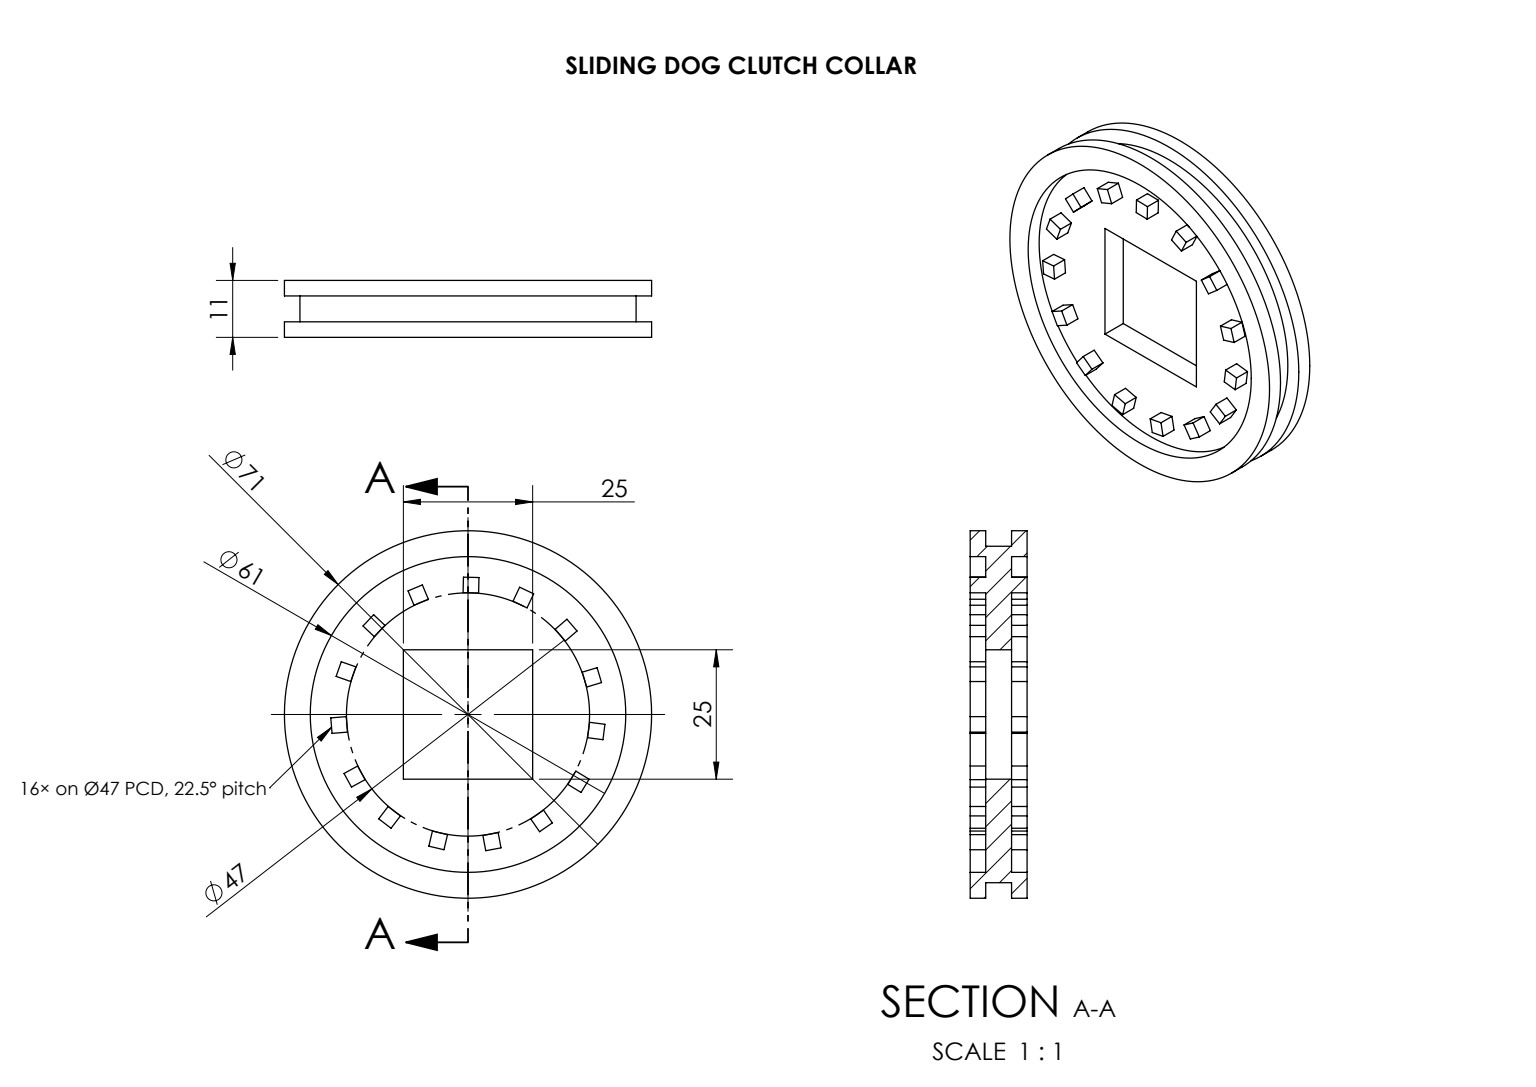
ISO-10303-21;
HEADER;
FILE_DESCRIPTION (('STEP AP214'),
    '1' );
FILE_NAME ('Sliding Dog Clutch Collar.step',
    '2026-09-30T12:41:04',
    ( '' ),
    ( '' ),
    'SwSTEP 2.0',
    'SolidWorks 2026',
    '' );
FILE_SCHEMA (( 'AUTOMOTIVE_DESIGN' ));
ENDSEC;

DATA;
#8=ORIENTED_EDGE ( 'NONE', *, *, #47564, .F. ) ;
#9=CARTESIAN_POINT ( 'NONE',  ( 0.000000000000000000, -120.0000000000000000, -5.500000000000000000 ) ) ;
#30=DIRECTION ( 'NONE',  ( -0.6516173805718067369, 0.7585478161175716050, 0.000000000000000000 ) ) ;
#32=AXIS2_PLACEMENT_3D ( 'NONE', #39036, #42465, #12856 ) ;
#46=EDGE_CURVE ( 'NONE', #39583, #27608, #108, .T. ) ;
#61=VECTOR ( 'NONE', #12342, 1000.000000000000114 ) ;
#65=DIRECTION ( 'NONE',  ( 0.000000000000000000, 1.000000000000000000, 0.000000000000000000 ) ) ;
#66=DIRECTION ( 'NONE',  ( -0.000000000000000000, -0.000000000000000000, -1.000000000000000000 ) ) ;
#75=AXIS2_PLACEMENT_3D ( 'NONE', #43340, #46778, #40148 ) ;
#80=ORIENTED_EDGE ( 'NONE', *, *, #29393, .F. ) ;
#108=LINE ( 'NONE', #14814, #16119 ) ;
#110=FACE_OUTER_BOUND ( 'NONE', #38176, .T. ) ;
#122=CARTESIAN_POINT ( 'NONE',  ( 23.49916127795269460, -121.5130826919798039, -5.500000000000000000 ) ) ;
#149=ORIENTED_EDGE ( 'NONE', *, *, #40004, .F. ) ;
#160=EDGE_CURVE ( 'NONE', #47761, #19570, #831, .T. ) ;
#163=LINE ( 'NONE', #8479, #41980 ) ;
#164=DIRECTION ( 'NONE',  ( -0.9966891607226785466, -0.08130631524010122069, 0.000000000000000000 ) ) ;
#165=CARTESIAN_POINT ( 'NONE',  ( 9.984461079971730157, -95.40710393340120277, 5.500000000000000000 ) ) ;
#171=LINE ( 'NONE', #44725, #4221 ) ;
#173=AXIS2_PLACEMENT_3D ( 'NONE', #10404, #35866, #3285 ) ;
#181=ORIENTED_EDGE ( 'NONE', *, *, #17068, .F. ) ;
#187=EDGE_CURVE ( 'NONE', #17280, #1537, #37135, .T. ) ;
#211=CARTESIAN_POINT ( 'NONE',  ( 21.85433023846371370, -135.0628101570779620, 5.500000000000000000 ) ) ;
#212=CARTESIAN_POINT ( 'NONE',  ( 0.4301293587033142574, -121.4370068666438556, 2.500000000000000000 ) ) ;
#222=CARTESIAN_POINT ( 'NONE',  ( -8.826826895187510402, -94.96827758698185562, 5.500000000000000000 ) ) ;
#244=VECTOR ( 'NONE', #1818, 1000.000000000000114 ) ;
#254=EDGE_LOOP ( 'NONE', ( #41035, #46518, #11215, #569 ) ) ;
#256=VECTOR ( 'NONE', #6458, 1000.000000000000000 ) ;
#273=DIRECTION ( 'NONE',  ( -0.6064928550163533050, -0.7950889364178781449, 0.000000000000000000 ) ) ;
#283=DIRECTION ( 'NONE',  ( -0.3853207896976533764, 0.9227826878668546895, 0.000000000000000000 ) ) ;
#285=VECTOR ( 'NONE', #16064, 1000.000000000000114 ) ;
#296=VECTOR ( 'NONE', #11332, 1000.000000000000227 ) ;
#303=ORIENTED_EDGE ( 'NONE', *, *, #45962, .F. ) ;
#309=DIRECTION ( 'NONE',  ( 0.8774505977381978905, 0.4796670183876304283, 0.000000000000000000 ) ) ;
#324=VECTOR ( 'NONE', #48391, 1000.000000000000114 ) ;
#327=CARTESIAN_POINT ( 'NONE',  ( 21.07894319797337701, -103.8699611390234878, 5.500000000000000000 ) ) ;
#342=CARTESIAN_POINT ( 'NONE',  ( -12.50000000000000000, -107.5000000000000000, 2.500000000000000000 ) ) ;
#355=DIRECTION ( 'NONE',  ( 0.8541291221503275466, -0.5200609990132993854, 0.000000000000000000 ) ) ;
#370=CARTESIAN_POINT ( 'NONE',  ( 12.13205353604972991, -140.1820037904669789, 5.500000000000000000 ) ) ;
#385=ADVANCED_FACE ( 'NONE', ( #12022 ), #4437, .F. ) ;
#392=ORIENTED_EDGE ( 'NONE', *, *, #17689, .T. ) ;
#397=FACE_OUTER_BOUND ( 'NONE', #27506, .T. ) ;
#412=VECTOR ( 'NONE', #23395, 1000.000000000000000 ) ;
#446=CARTESIAN_POINT ( 'NONE',  ( -13.05994868825747446, -139.5943292883446532, 5.500000000000000000 ) ) ;
#448=DIRECTION ( 'NONE',  ( -0.000000000000000000, -0.000000000000000000, -1.000000000000000000 ) ) ;
#449=ORIENTED_EDGE ( 'NONE', *, *, #48116, .F. ) ;
#454=FACE_OUTER_BOUND ( 'NONE', #32688, .T. ) ;
#459=VECTOR ( 'NONE', #14578, 1000.000000000000114 ) ;
#460=ORIENTED_EDGE ( 'NONE', *, *, #19536, .T. ) ;
#473=DIRECTION ( 'NONE',  ( -0.000000000000000000, -0.000000000000000000, -1.000000000000000000 ) ) ;
#474=ORIENTED_EDGE ( 'NONE', *, *, #31629, .F. ) ;
#480=PLANE ( 'NONE',  #23178 ) ;
#482=ORIENTED_EDGE ( 'NONE', *, *, #3297, .T. ) ;
#494=LINE ( 'NONE', #44786, #14354 ) ;
#509=FACE_OUTER_BOUND ( 'NONE', #15713, .T. ) ;
#513=ORIENTED_EDGE ( 'NONE', *, *, #3767, .F. ) ;
#537=DIRECTION ( 'NONE',  ( -0.9730327541852497042, 0.2306669878475622604, 0.000000000000000000 ) ) ;
#542=DIRECTION ( 'NONE',  ( -0.000000000000000000, -0.000000000000000000, -1.000000000000000000 ) ) ;
#544=DIRECTION ( 'NONE',  ( 0.9918136447140100120, -0.1276937514489704939, 0.000000000000000000 ) ) ;
#551=VERTEX_POINT ( 'NONE', #27927 ) ;
#555=EDGE_CURVE ( 'NONE', #16750, #43974, #5886, .T. ) ;
#567=LINE ( 'NONE', #45118, #45725 ) ;
#569=ORIENTED_EDGE ( 'NONE', *, *, #23324, .F. ) ;
#570=CARTESIAN_POINT ( 'NONE',  ( 16.30584220631899228, -140.9432449716519784, 5.500000000000000000 ) ) ;
#571=CARTESIAN_POINT ( 'NONE',  ( 1.029419772574596825, -118.9089936151275140, 2.500000000000000000 ) ) ;
#576=ORIENTED_EDGE ( 'NONE', *, *, #44143, .F. ) ;
#594=LINE ( 'NONE', #15524, #29851 ) ;
#598=CARTESIAN_POINT ( 'NONE',  ( 4.903647372192503795, -146.0423547792665886, 2.500000000000000000 ) ) ;
#601=CARTESIAN_POINT ( 'NONE',  ( 20.85212586905262100, -130.9402397935870965, 5.500000000000000000 ) ) ;
#622=EDGE_LOOP ( 'NONE', ( #38651, #1089, #2965, #8815 ) ) ;
#639=PLANE ( 'NONE',  #10239 ) ;
#656=PLANE ( 'NONE',  #42750 ) ;
#669=ORIENTED_EDGE ( 'NONE', *, *, #7293, .T. ) ;
#693=PLANE ( 'NONE',  #5618 ) ;
#722=LINE ( 'NONE', #11518, #33116 ) ;
#724=ORIENTED_EDGE ( 'NONE', *, *, #41620, .T. ) ;
#730=CARTESIAN_POINT ( 'NONE',  ( 20.85212586905262100, -130.9402397935870965, 2.500000000000000000 ) ) ;
#733=CARTESIAN_POINT ( 'NONE',  ( -23.30023580412278505, -123.4057321492263384, -5.500000000000000000 ) ) ;
#741=FACE_OUTER_BOUND ( 'NONE', #31676, .T. ) ;
#744=ORIENTED_EDGE ( 'NONE', *, *, #10469, .F. ) ;
#748=CARTESIAN_POINT ( 'NONE',  ( -7.572224309238338336, -145.4393675041377492, 5.500000000000000000 ) ) ;
#756=EDGE_CURVE ( 'NONE', #40958, #16750, #45009, .T. ) ;
#769=CARTESIAN_POINT ( 'NONE',  ( -13.05994868825747446, -139.5943292883446532, 5.500000000000000000 ) ) ;
#781=EDGE_LOOP ( 'NONE', ( #17034, #22607, #22558, #21129 ) ) ;
#792=CARTESIAN_POINT ( 'NONE',  ( 0.1219594728601484379, -121.4950337410840149, 2.500000000000000000 ) ) ;
#831=LINE ( 'NONE', #10898, #11447 ) ;
#864=CARTESIAN_POINT ( 'NONE',  ( -14.87942725330654348, -141.9795960975983178, 5.500000000000000000 ) ) ;
#866=LINE ( 'NONE', #30749, #3355 ) ;
#877=AXIS2_PLACEMENT_3D ( 'NONE', #15679, #17351, #43081 ) ;
#896=CARTESIAN_POINT ( 'NONE',  ( -10.43921258969510824, -98.89258801967538659, 5.500000000000000000 ) ) ;
#906=DIRECTION ( 'NONE',  ( 0.5200609990133008287, 0.8541291221503266584, -0.000000000000000000 ) ) ;
#935=CARTESIAN_POINT ( 'NONE',  ( -15.44521549751111422, -137.7748507232956001, 2.500000000000000000 ) ) ;
#974=VECTOR ( 'NONE', #38147, 1000.000000000000000 ) ;
#1021=CARTESIAN_POINT ( 'NONE',  ( 19.29194287201271862, -133.5026271600380880, -5.500000000000000000 ) ) ;
#1026=DIRECTION ( 'NONE',  ( -0.000000000000000000, -0.000000000000000000, -1.000000000000000000 ) ) ;
#1068=VECTOR ( 'NONE', #42092, 1000.000000000000000 ) ;
#1072=VECTOR ( 'NONE', #42654, 1000.000000000000000 ) ;
#1074=ORIENTED_EDGE ( 'NONE', *, *, #30261, .F. ) ;
#1087=ADVANCED_FACE ( 'NONE', ( #43978, #17297, #32251, #21211, #40330, #14365, #36627, #36147, #6784, #21706, #21939, #17545, #3091, #47414, #18018, #47170, #44228 ), #2603, .F. ) ;
#1089=ORIENTED_EDGE ( 'NONE', *, *, #1604, .T. ) ;
#1090=EDGE_CURVE ( 'NONE', #29594, #25561, #7011, .T. ) ;
#1103=ADVANCED_FACE ( 'NONE', ( #30272 ), #41519, .T. ) ;
#1105=CARTESIAN_POINT ( 'NONE',  ( -1.459549131277904976, -119.6539995182286304, 2.500000000000000000 ) ) ;
#1110=DIRECTION ( 'NONE',  ( 0.9997280174009349762, -0.02332147558787674158, 0.000000000000000000 ) ) ;
#1113=CARTESIAN_POINT ( 'NONE',  ( 2.874421927457452952, -143.3717286177755739, 5.500000000000000000 ) ) ;
#1124=AXIS2_PLACEMENT_3D ( 'NONE', #13235, #28158, #27444 ) ;
#1129=AXIS2_PLACEMENT_3D ( 'NONE', #7232, #11155, #3564 ) ;
#1132=VECTOR ( 'NONE', #38496, 1000.000000000000000 ) ;
#1140=ORIENTED_EDGE ( 'NONE', *, *, #8337, .F. ) ;
#1141=AXIS2_PLACEMENT_3D ( 'NONE', #1935, #20508, #43039 ) ;
#1148=EDGE_CURVE ( 'NONE', #30085, #18493, #4073, .T. ) ;
#1152=ORIENTED_EDGE ( 'NONE', *, *, #6211, .T. ) ;
#1157=AXIS2_PLACEMENT_3D ( 'NONE', #25787, #14062, #26038 ) ;
#1176=DIRECTION ( 'NONE',  ( 0.8774505977381983346, 0.4796670183876293736, 0.000000000000000000 ) ) ;
#1190=ORIENTED_EDGE ( 'NONE', *, *, #32089, .F. ) ;
#1204=FACE_OUTER_BOUND ( 'NONE', #23258, .T. ) ;
#1206=AXIS2_PLACEMENT_3D ( 'NONE', #14979, #37488, #45543 ) ;
#1207=CARTESIAN_POINT ( 'NONE',  ( 21.07894319797337701, -103.8699611390234878, -5.500000000000000000 ) ) ;
#1210=ORIENTED_EDGE ( 'NONE', *, *, #1703, .T. ) ;
#1221=ORIENTED_EDGE ( 'NONE', *, *, #12348, .F. ) ;
#1232=VECTOR ( 'NONE', #47384, 1000.000000000000000 ) ;
#1269=PLANE ( 'NONE',  #48175 ) ;
#1339=ADVANCED_FACE ( 'NONE', ( #12388 ), #35368, .F. ) ;
#1355=VECTOR ( 'NONE', #38110, 1000.000000000000000 ) ;
#1356=PLANE ( 'NONE',  #32 ) ;
#1361=DIRECTION ( 'NONE',  ( -0.9997280174009349762, 0.02332147558787674504, 0.000000000000000000 ) ) ;
#1382=ORIENTED_EDGE ( 'NONE', *, *, #44642, .T. ) ;
#1391=VECTOR ( 'NONE', #38209, 1000.000000000000000 ) ;
#1422=ORIENTED_EDGE ( 'NONE', *, *, #10339, .F. ) ;
#1444=DIRECTION ( 'NONE',  ( 0.4796670183876317051, -0.8774505977381971134, 0.000000000000000000 ) ) ;
#1451=DIRECTION ( 'NONE',  ( 0.2867529058022035837, -0.9580045777625452175, 0.000000000000000000 ) ) ;
#1453=LINE ( 'NONE', #23715, #23723 ) ;
#1454=SURFACE_STYLE_FILL_AREA ( #43295 ) ;
#1456=EDGE_CURVE ( 'NONE', #36858, #6225, #7138, .T. ) ;
#1478=FACE_OUTER_BOUND ( 'NONE', #8267, .T. ) ;
#1489=AXIS2_PLACEMENT_3D ( 'NONE', #7046, #21739, #18554 ) ;
#1496=DIRECTION ( 'NONE',  ( -0.7273375899149802093, 0.6862798483830544471, 0.000000000000000000 ) ) ;
#1499=VECTOR ( 'NONE', #43191, 1000.000000000000114 ) ;
#1502=LINE ( 'NONE', #45547, #9467 ) ;
#1517=ADVANCED_FACE ( 'NONE', ( #32830 ), #36744, .F. ) ;
#1520=DIRECTION ( 'NONE',  ( 0.9435911131814398445, -0.3311129884571295534, 0.000000000000000000 ) ) ;
#1537=VERTEX_POINT ( 'NONE', #38212 ) ;
#1541=FACE_OUTER_BOUND ( 'NONE', #34357, .T. ) ;
#1542=LINE ( 'NONE', #45859, #18896 ) ;
#1567=CARTESIAN_POINT ( 'NONE',  ( 23.49916127795269460, -121.5130826919798039, 5.500000000000000000 ) ) ;
#1596=CARTESIAN_POINT ( 'NONE',  ( -1.355716935723729089, -119.3581031311870362, 2.500000000000000000 ) ) ;
#1597=VECTOR ( 'NONE', #34107, 1000.000000000000114 ) ;
#1600=ORIENTED_EDGE ( 'NONE', *, *, #21124, .F. ) ;
#1604=EDGE_CURVE ( 'NONE', #10011, #41264, #23755, .T. ) ;
#1605=CARTESIAN_POINT ( 'NONE',  ( -18.12185313557660038, -104.9634299478706794, -5.500000000000000000 ) ) ;
#1610=EDGE_CURVE ( 'NONE', #42762, #16099, #26471, .T. ) ;
#1613=VERTEX_POINT ( 'NONE', #12036 ) ;
#1620=EDGE_CURVE ( 'NONE', #25900, #44934, #41405, .T. ) ;
#1621=CARTESIAN_POINT ( 'NONE',  ( -18.24502636017239965, -100.7225776329765665, 2.500000000000000000 ) ) ;
#1626=CARTESIAN_POINT ( 'NONE',  ( 6.377742925735834234, -145.7647898336708181, 5.500000000000000000 ) ) ;
#1632=VECTOR ( 'NONE', #39657, 1000.000000000000114 ) ;
#1639=LINE ( 'NONE', #5552, #36656 ) ;
#1642=LINE ( 'NONE', #12423, #39045 ) ;
#1643=DIRECTION ( 'NONE',  ( -0.8541291221503265474, 0.5200609990133007177, 0.000000000000000000 ) ) ;
#1648=CARTESIAN_POINT ( 'NONE',  ( 1.384174031800307736, -119.4220188154534981, 2.500000000000000000 ) ) ;
#1654=ORIENTED_EDGE ( 'NONE', *, *, #12136, .T. ) ;
#1656=ORIENTED_EDGE ( 'NONE', *, *, #27421, .F. ) ;
#1667=ORIENTED_EDGE ( 'NONE', *, *, #7528, .F. ) ;
#1673=DIRECTION ( 'NONE',  ( 0.3853207896976523772, -0.9227826878668550226, 0.000000000000000000 ) ) ;
#1681=DIRECTION ( 'NONE',  ( -0.6516173805718079581, 0.7585478161175704948, 0.000000000000000000 ) ) ;
#1703=EDGE_CURVE ( 'NONE', #37836, #30905, #10029, .T. ) ;
#1712=ADVANCED_FACE ( 'NONE', ( #9790 ), #1731, .T. ) ;
#1714=ORIENTED_EDGE ( 'NONE', *, *, #46087, .F. ) ;
#1731=PLANE ( 'NONE',  #26803 ) ;
#1734=FACE_OUTER_BOUND ( 'NONE', #37102, .T. ) ;
#1738=VECTOR ( 'NONE', #7203, 1000.000000000000227 ) ;
#1747=EDGE_LOOP ( 'NONE', ( #24600, #3735, #14159, #36604 ) ) ;
#1753=CARTESIAN_POINT ( 'NONE',  ( 2.117611129180199558, -93.54218975225703048, 5.500000000000000000 ) ) ;
#1755=CARTESIAN_POINT ( 'NONE',  ( -20.30386590532152979, -102.9045904027214959, 5.500000000000000000 ) ) ;
#1759=EDGE_CURVE ( 'NONE', #4190, #39318, #42854, .T. ) ;
#1778=PLANE ( 'NONE',  #23131 ) ;
#1785=ORIENTED_EDGE ( 'NONE', *, *, #39352, .F. ) ;
#1801=VECTOR ( 'NONE', #34768, 1000.000000000000114 ) ;
#1818=DIRECTION ( 'NONE',  ( 0.9918136447140101231, -0.1276937514489694114, 0.000000000000000000 ) ) ;
#1834=FACE_OUTER_BOUND ( 'NONE', #20477, .T. ) ;
#1861=CARTESIAN_POINT ( 'NONE',  ( 8.700667342345820288, -98.11853780484867116, -5.500000000000000000 ) ) ;
#1874=VERTEX_POINT ( 'NONE', #10997 ) ;
#1887=ADVANCED_FACE ( 'NONE', ( #10760 ), #40854, .T. ) ;
#1888=VECTOR ( 'NONE', #1643, 1000.000000000000227 ) ;
#1892=ORIENTED_EDGE ( 'NONE', *, *, #43418, .T. ) ;
#1897=EDGE_LOOP ( 'NONE', ( #30604, #10445, #36560, #36897 ) ) ;
#1920=VECTOR ( 'NONE', #32364, 1000.000000000000114 ) ;
#1935=CARTESIAN_POINT ( 'NONE',  ( 0.000000000000000000, -120.0000000000000000, 2.500000000000000000 ) ) ;
#1947=EDGE_LOOP ( 'NONE', ( #17212, #46442, #44132, #37392 ) ) ;
#1949=ADVANCED_FACE ( 'NONE', ( #25429 ), #21761, .F. ) ;
#1956=ORIENTED_EDGE ( 'NONE', *, *, #26185, .F. ) ;
#1965=ORIENTED_EDGE ( 'NONE', *, *, #17987, .F. ) ;
#1985=CARTESIAN_POINT ( 'NONE',  ( 9.984461079971730157, -95.40710393340120277, 5.500000000000000000 ) ) ;
#1992=PLANE ( 'NONE',  #5433 ) ;
#1998=DIRECTION ( 'NONE',  ( -0.6516173805718079581, 0.7585478161175704948, 0.000000000000000000 ) ) ;
#2010=LINE ( 'NONE', #12532, #5745 ) ;
#2021=ORIENTED_EDGE ( 'NONE', *, *, #1620, .F. ) ;
#2034=CARTESIAN_POINT ( 'NONE',  ( 3.429551818649054340, -146.3199197248623875, 5.500000000000000000 ) ) ;
#2037=CARTESIAN_POINT ( 'NONE',  ( 9.984461079971730157, -95.40710393340121698, -2.500000000000000000 ) ) ;
#2048=ORIENTED_EDGE ( 'NONE', *, *, #26203, .T. ) ;
#2053=DIRECTION ( 'NONE',  ( 0.9038112904824853189, -0.4279312458752977388, 0.000000000000000000 ) ) ;
#2058=DIRECTION ( 'NONE',  ( -0.000000000000000000, -0.000000000000000000, -1.000000000000000000 ) ) ;
#2059=EDGE_CURVE ( 'NONE', #47361, #20756, #22975, .T. ) ;
#2065=CARTESIAN_POINT ( 'NONE',  ( 26.09152095774781799, -124.8716048804687375, 5.500000000000000000 ) ) ;
#2067=CARTESIAN_POINT ( 'NONE',  ( -0.1219594728601508804, -118.5049662589159567, 2.500000000000000000 ) ) ;
#2070=ORIENTED_EDGE ( 'NONE', *, *, #39079, .T. ) ;
#2081=DIRECTION ( 'NONE',  ( -0.7585478161175706058, -0.6516173805718078471, 0.000000000000000000 ) ) ;
#2086=CARTESIAN_POINT ( 'NONE',  ( 2.117611129180199558, -93.54218975225703048, -5.500000000000000000 ) ) ;
#2092=DIRECTION ( 'NONE',  ( -0.9730327541852497042, 0.2306669878475623159, 0.000000000000000000 ) ) ;
#2102=CARTESIAN_POINT ( 'NONE',  ( -6.112675177960399608, -145.7853679859090903, -2.500000000000000000 ) ) ;
#2105=VECTOR ( 'NONE', #1681, 1000.000000000000114 ) ;
#2113=CARTESIAN_POINT ( 'NONE',  ( -4.653126046682595884, -146.1313684676804314, -5.500000000000000000 ) ) ;
#2150=LINE ( 'NONE', #35423, #18106 ) ;
#2155=ORIENTED_EDGE ( 'NONE', *, *, #14480, .T. ) ;
#2158=VERTEX_POINT ( 'NONE', #16363 ) ;
#2170=ORIENTED_EDGE ( 'NONE', *, *, #24897, .F. ) ;
#2193=ORIENTED_EDGE ( 'NONE', *, *, #28126, .F. ) ;
#2202=ORIENTED_EDGE ( 'NONE', *, *, #6000, .F. ) ;
#2209=DIRECTION ( 'NONE',  ( 0.6691306063588671194, -0.7431448254773862505, 0.000000000000000000 ) ) ;
#2213=DIRECTION ( 'NONE',  ( 0.000000000000000000, 0.000000000000000000, 1.000000000000000000 ) ) ;
#2218=FACE_OUTER_BOUND ( 'NONE', #45782, .T. ) ;
#2223=CARTESIAN_POINT ( 'NONE',  ( -8.826826895187510402, -94.96827758698185562, 5.500000000000000000 ) ) ;
#2249=AXIS2_PLACEMENT_3D ( 'NONE', #29811, #906, #18783 ) ;
#2251=EDGE_CURVE ( 'NONE', #46736, #9579, #39845, .T. ) ;
#2278=ORIENTED_EDGE ( 'NONE', *, *, #16209, .F. ) ;
#2285=ORIENTED_EDGE ( 'NONE', *, *, #17271, .F. ) ;
#2298=EDGE_CURVE ( 'NONE', #34199, #30446, #21715, .T. ) ;
#2300=ORIENTED_EDGE ( 'NONE', *, *, #35031, .F. ) ;
#2301=DIRECTION ( 'NONE',  ( 0.6862798483830554463, 0.7273375899149793211, -0.000000000000000000 ) ) ;
#2318=LINE ( 'NONE', #46395, #15226 ) ;
#2333=LINE ( 'NONE', #21415, #40946 ) ;
#2344=ORIENTED_EDGE ( 'NONE', *, *, #17071, .F. ) ;
#2349=AXIS2_PLACEMENT_3D ( 'NONE', #29628, #14221, #36491 ) ;
#2353=DIRECTION ( 'NONE',  ( -0.9435911131814395114, 0.3311129884571304971, 0.000000000000000000 ) ) ;
#2356=EDGE_LOOP ( 'NONE', ( #8, #42729, #13824, #11043 ) ) ;
#2358=ORIENTED_EDGE ( 'NONE', *, *, #26413, .T. ) ;
#2360=CARTESIAN_POINT ( 'NONE',  ( 25.81725066941077884, -113.8380548628854854, 2.500000000000000000 ) ) ;
#2361=DIRECTION ( 'NONE',  ( -0.9918136447140101231, 0.1276937514489694114, 0.000000000000000000 ) ) ;
#2372=ADVANCED_FACE ( 'NONE', ( #30511 ), #30031, .F. ) ;
#2378=VECTOR ( 'NONE', #21321, 999.9999999999998863 ) ;
#2403=VECTOR ( 'NONE', #44413, 999.9999999999998863 ) ;
#2423=VERTEX_POINT ( 'NONE', #16075 ) ;
#2436=ORIENTED_EDGE ( 'NONE', *, *, #42893, .T. ) ;
#2478=PLANE ( 'NONE',  #10175 ) ;
#2490=CARTESIAN_POINT ( 'NONE',  ( 12.69589495141918611, -96.69089767102708777, 2.500000000000000000 ) ) ;
#2495=CARTESIAN_POINT ( 'NONE',  ( -24.50849501662245800, -109.8101191361138831, 5.500000000000000000 ) ) ;
#2510=CARTESIAN_POINT ( 'NONE',  ( 12.50000000000000000, -107.5000000000000000, -2.500000000000000000 ) ) ;
#2525=ORIENTED_EDGE ( 'NONE', *, *, #41936, .F. ) ;
#2527=LINE ( 'NONE', #25282, #256 ) ;
#2538=ORIENTED_EDGE ( 'NONE', *, *, #20611, .F. ) ;
#2542=VECTOR ( 'NONE', #33099, 1000.000000000000000 ) ;
#2551=CARTESIAN_POINT ( 'NONE',  ( -22.67106064244953245, -113.6342314410295842, -5.500000000000000000 ) ) ;
#2590=AXIS2_PLACEMENT_3D ( 'NONE', #34307, #26996, #27229 ) ;
#2603=PLANE ( 'NONE',  #12776 ) ;
#2624=CARTESIAN_POINT ( 'NONE',  ( 21.07894319797337701, -103.8699611390234878, -5.500000000000000000 ) ) ;
#2641=EDGE_CURVE ( 'NONE', #5936, #21061, #40510, .T. ) ;
#2642=VECTOR ( 'NONE', #33467, 1000.000000000000000 ) ;
#2644=VECTOR ( 'NONE', #21822, 1000.000000000000000 ) ;
#2655=AXIS2_PLACEMENT_3D ( 'NONE', #21959, #10953, #11198 ) ;
#2739=ORIENTED_EDGE ( 'NONE', *, *, #29724, .T. ) ;
#2780=CARTESIAN_POINT ( 'NONE',  ( -70.53423027509626309, -217.0820393249940423, 5.500000000000000000 ) ) ;
#2789=DIRECTION ( 'NONE',  ( 0.5687579148473743684, -0.8225049752423791993, 0.000000000000000000 ) ) ;
#2791=LINE ( 'NONE', #47102, #30618 ) ;
#2793=VERTEX_POINT ( 'NONE', #33631 ) ;
#2795=VERTEX_POINT ( 'NONE', #12111 ) ;
#2808=EDGE_CURVE ( 'NONE', #4369, #29100, #594, .T. ) ;
#2834=ADVANCED_FACE ( 'NONE', ( #27764 ), #5244, .F. ) ;
#2839=LINE ( 'NONE', #37339, #27728 ) ;
#2880=DIRECTION ( 'NONE',  ( 0.9918136447140100120, -0.1276937514489704939, 0.000000000000000000 ) ) ;
#2884=CARTESIAN_POINT ( 'NONE',  ( -24.50849501662245800, -109.8101191361138831, 5.500000000000000000 ) ) ;
#2897=ORIENTED_EDGE ( 'NONE', *, *, #43439, .T. ) ;
#2919=VECTOR ( 'NONE', #4815, 1000.000000000000000 ) ;
#2927=CARTESIAN_POINT ( 'NONE',  ( 35.50000000000000711, -120.0000000000000000, 5.500000000000000000 ) ) ;
#2942=VERTEX_POINT ( 'NONE', #10105 ) ;
#2960=EDGE_CURVE ( 'NONE', #13263, #35674, #13535, .T. ) ;
#2962=EDGE_LOOP ( 'NONE', ( #38495, #17345, #23916, #2155 ) ) ;
#2965=ORIENTED_EDGE ( 'NONE', *, *, #42796, .T. ) ;
#2984=VECTOR ( 'NONE', #9958, 1000.000000000000227 ) ;
#2994=CARTESIAN_POINT ( 'NONE',  ( 26.09152095774781799, -124.8716048804687375, 5.500000000000000000 ) ) ;
#3000=ORIENTED_EDGE ( 'NONE', *, *, #17073, .F. ) ;
#3014=VECTOR ( 'NONE', #38561, 1000.000000000000000 ) ;
#3041=DIRECTION ( 'NONE',  ( -0.9038112904824846527, 0.4279312458752990711, 0.000000000000000000 ) ) ;
#3064=EDGE_LOOP ( 'NONE', ( #41739, #6003, #17795, #31442 ) ) ;
#3082=ORIENTED_EDGE ( 'NONE', *, *, #32089, .T. ) ;
#3090=ADVANCED_FACE ( 'NONE', ( #7401 ), #18414, .F. ) ;
#3091=FACE_BOUND ( 'NONE', #16469, .T. ) ;
#3101=CARTESIAN_POINT ( 'NONE',  ( 2.047646702416564324, -96.54137380445985173, -2.500000000000000000 ) ) ;
#3104=FACE_OUTER_BOUND ( 'NONE', #18786, .T. ) ;
#3107=CARTESIAN_POINT ( 'NONE',  ( -22.67106064244953245, -113.6342314410295842, 5.500000000000000000 ) ) ;
#3108=FACE_OUTER_BOUND ( 'NONE', #37345, .T. ) ;
#3111=CARTESIAN_POINT ( 'NONE',  ( -22.67106064244953245, -113.6342314410295842, -5.500000000000000000 ) ) ;
#3116=ORIENTED_EDGE ( 'NONE', *, *, #17112, .T. ) ;
#3130=LINE ( 'NONE', #21517, #42294 ) ;
#3152=DIRECTION ( 'NONE',  ( -0.4279312458752977388, -0.9038112904824853189, 0.000000000000000000 ) ) ;
#3158=LINE ( 'NONE', #31860, #9695 ) ;
#3188=VERTEX_POINT ( 'NONE', #30168 ) ;
#3198=EDGE_LOOP ( 'NONE', ( #11283, #46464, #34828, #29564 ) ) ;
#3205=ORIENTED_EDGE ( 'NONE', *, *, #22373, .F. ) ;
#3228=AXIS2_PLACEMENT_3D ( 'NONE', #24463, #39408, #5389 ) ;
#3234=VERTEX_POINT ( 'NONE', #3480 ) ;
#3255=EDGE_CURVE ( 'NONE', #9902, #23423, #32264, .T. ) ;
#3263=LINE ( 'NONE', #18188, #1499 ) ;
#3269=ORIENTED_EDGE ( 'NONE', *, *, #19805, .T. ) ;
#3285=DIRECTION ( 'NONE',  ( 0.3090169943749448977, 0.9510565162951543083, 0.000000000000000000 ) ) ;
#3288=CARTESIAN_POINT ( 'NONE',  ( 5.822613034544236399, -142.8165987265839760, 5.500000000000000000 ) ) ;
#3291=ORIENTED_EDGE ( 'NONE', *, *, #19897, .F. ) ;
#3297=EDGE_CURVE ( 'NONE', #12549, #23907, #38899, .T. ) ;
#3299=EDGE_CURVE ( 'NONE', #12589, #8139, #6088, .T. ) ;
#3314=ORIENTED_EDGE ( 'NONE', *, *, #16929, .F. ) ;
#3323=ADVANCED_FACE ( 'NONE', ( #3104 ), #29789, .F. ) ;
#3324=FACE_BOUND ( 'NONE', #22303, .T. ) ;
#3348=DIRECTION ( 'NONE',  ( -0.3853207896976523772, 0.9227826878668550226, 0.000000000000000000 ) ) ;
#3354=ADVANCED_FACE ( 'NONE', ( #41071 ), #40568, .F. ) ;
#3355=VECTOR ( 'NONE', #28045, 1000.000000000000000 ) ;
#3358=CARTESIAN_POINT ( 'NONE',  ( 2.047646702416564768, -96.54137380445985173, 5.500000000000000000 ) ) ;
#3365=ORIENTED_EDGE ( 'NONE', *, *, #11147, .T. ) ;
#3369=CARTESIAN_POINT ( 'NONE',  ( -10.43921258969510824, -98.89258801967538659, 5.500000000000000000 ) ) ;
#3370=VERTEX_POINT ( 'NONE', #17805 ) ;
#3371=ORIENTED_EDGE ( 'NONE', *, *, #23331, .F. ) ;
#3387=DIRECTION ( 'NONE',  ( 0.1276937514489694392, 0.9918136447140102341, -0.000000000000000000 ) ) ;
#3392=AXIS2_PLACEMENT_3D ( 'NONE', #8353, #42368, #12040 ) ;
#3413=LINE ( 'NONE', #36474, #3701 ) ;
#3429=AXIS2_PLACEMENT_3D ( 'NONE', #211, #44529, #15170 ) ;
#3432=ORIENTED_EDGE ( 'NONE', *, *, #11070, .T. ) ;
#3440=AXIS2_PLACEMENT_3D ( 'NONE', #11817, #26748, #7431 ) ;
#3456=FACE_OUTER_BOUND ( 'NONE', #6651, .T. ) ;
#3468=FACE_OUTER_BOUND ( 'NONE', #36043, .T. ) ;
#3472=EDGE_CURVE ( 'NONE', #9793, #9902, #44971, .T. ) ;
#3480=CARTESIAN_POINT ( 'NONE',  ( 23.11608002360578240, -124.4885236261218182, 2.500000000000000000 ) ) ;
#3499=DIRECTION ( 'NONE',  ( -0.000000000000000000, -0.000000000000000000, -1.000000000000000000 ) ) ;
#3501=EDGE_CURVE ( 'NONE', #24269, #29100, #163, .T. ) ;
#3504=EDGE_LOOP ( 'NONE', ( #5725, #7666, #12034, #15312 ) ) ;
#3507=LINE ( 'NONE', #37284, #15629 ) ;
#3514=CARTESIAN_POINT ( 'NONE',  ( -0.8815729230226008184, -93.47222532549339746, -5.500000000000000000 ) ) ;
#3523=CARTESIAN_POINT ( 'NONE',  ( -7.572224309238338336, -145.4393675041377492, -5.500000000000000000 ) ) ;
#3524=ADVANCED_FACE ( 'NONE', ( #11453 ), #45213, .T. ) ;
#3533=LINE ( 'NONE', #18465, #6307 ) ;
#3544=ADVANCED_FACE ( 'NONE', ( #34405 ), #656, .F. ) ;
#3546=VECTOR ( 'NONE', #13274, 1000.000000000000000 ) ;
#3548=DIRECTION ( 'NONE',  ( -0.9580045777625459946, -0.2867529058022011412, 0.000000000000000000 ) ) ;
#3564=DIRECTION ( 'NONE',  ( -0.2867529058022035837, 0.9580045777625452175, 0.000000000000000000 ) ) ;
#3571=VERTEX_POINT ( 'NONE', #45688 ) ;
#3578=ORIENTED_EDGE ( 'NONE', *, *, #33962, .T. ) ;
#3581=CARTESIAN_POINT ( 'NONE',  ( 35.50000000000000711, -120.0000000000000000, -2.500000000000000000 ) ) ;
#3610=DIRECTION ( 'NONE',  ( -0.9827303690289285187, -0.1850432970638656860, 0.000000000000000000 ) ) ;
#3616=ADVANCED_FACE ( 'NONE', ( #20702 ), #39069, .T. ) ;
#3644=ORIENTED_EDGE ( 'NONE', *, *, #15798, .T. ) ;
#3645=CARTESIAN_POINT ( 'NONE',  ( 18.80329974962065265, -105.8248132807389084, 5.500000000000000000 ) ) ;
#3647=VECTOR ( 'NONE', #14616, 1000.000000000000114 ) ;
#3655=DIRECTION ( 'NONE',  ( -0.5687579148473752566, 0.8225049752423786442, 0.000000000000000000 ) ) ;
#3662=VECTOR ( 'NONE', #12582, 1000.000000000000000 ) ;
#3667=DIRECTION ( 'NONE',  ( 1.000000000000000000, 0.000000000000000000, 0.000000000000000000 ) ) ;
#3668=CARTESIAN_POINT ( 'NONE',  ( 1.459549131277868561, -120.3460004817713411, -2.500000000000000000 ) ) ;
#3677=ORIENTED_EDGE ( 'NONE', *, *, #7779, .F. ) ;
#3679=AXIS2_PLACEMENT_3D ( 'NONE', #32431, #20196, #46390 ) ;
#3683=VECTOR ( 'NONE', #7084, 1000.000000000000000 ) ;
#3684=VERTEX_POINT ( 'NONE', #43220 ) ;
#3694=VERTEX_POINT ( 'NONE', #9931 ) ;
#3700=CARTESIAN_POINT ( 'NONE',  ( 20.10151712711562766, -102.7321394148470830, -2.500000000000000000 ) ) ;
#3701=VECTOR ( 'NONE', #44781, 1000.000000000000000 ) ;
#3706=DIRECTION ( 'NONE',  ( -0.8541291221503261033, 0.5200609990133016058, 0.000000000000000000 ) ) ;
#3720=EDGE_LOOP ( 'NONE', ( #10458, #47860, #46613, #20728 ) ) ;
#3727=LINE ( 'NONE', #44842, #17389 ) ;
#3731=EDGE_LOOP ( 'NONE', ( #45449, #16266, #35435, #23257 ) ) ;
#3733=DIRECTION ( 'NONE',  ( 0.9730327541852497042, -0.2306669878475622604, 0.000000000000000000 ) ) ;
#3735=ORIENTED_EDGE ( 'NONE', *, *, #17068, .T. ) ;
#3751=VECTOR ( 'NONE', #46897, 1000.000000000000000 ) ;
#3754=VECTOR ( 'NONE', #38869, 1000.000000000000114 ) ;
#3767=EDGE_CURVE ( 'NONE', #16750, #16956, #36822, .T. ) ;
#3785=FACE_OUTER_BOUND ( 'NONE', #20250, .T. ) ;
#3796=EDGE_CURVE ( 'NONE', #23423, #11302, #25805, .T. ) ;
#3803=ORIENTED_EDGE ( 'NONE', *, *, #1610, .F. ) ;
#3804=EDGE_CURVE ( 'NONE', #37452, #25110, #29000, .T. ) ;
#3805=AXIS2_PLACEMENT_3D ( 'NONE', #31386, #47016, #13481 ) ;
#3831=DIRECTION ( 'NONE',  ( -0.2306669878475637314, -0.9730327541852493711, 0.000000000000000000 ) ) ;
#3838=ADVANCED_FACE ( 'NONE', ( #32453 ), #7214, .F. ) ;
#3846=DIRECTION ( 'NONE',  ( 0.8225049752423776450, 0.5687579148473765889, 0.000000000000000000 ) ) ;
#3876=LINE ( 'NONE', #45004, #30961 ) ;
#3911=ORIENTED_EDGE ( 'NONE', *, *, #8358, .F. ) ;
#3914=EDGE_CURVE ( 'NONE', #10647, #20850, #45624, .T. ) ;
#3915=DIRECTION ( 'NONE',  ( 0.000000000000000000, 0.000000000000000000, 1.000000000000000000 ) ) ;
#3931=CARTESIAN_POINT ( 'NONE',  ( -0.7800914985199643992, -121.2811936832255100, -2.500000000000000000 ) ) ;
#3942=CARTESIAN_POINT ( 'NONE',  ( 2.874421927457452952, -143.3717286177755739, 5.500000000000000000 ) ) ;
#3950=EDGE_CURVE ( 'NONE', #14358, #28358, #44905, .T. ) ;
#3981=ADVANCED_FACE ( 'NONE', ( #11390 ), #30463, .F. ) ;
#3984=VECTOR ( 'NONE', #1673, 1000.000000000000114 ) ;
#4005=AXIS2_PLACEMENT_3D ( 'NONE', #36683, #3387, #18330 ) ;
#4011=EDGE_LOOP ( 'NONE', ( #1714, #11285, #46389, #35520 ) ) ;
#4016=ORIENTED_EDGE ( 'NONE', *, *, #44597, .T. ) ;
#4019=LINE ( 'NONE', #26040, #1597 ) ;
#4052=DIRECTION ( 'NONE',  ( -0.000000000000000000, -0.000000000000000000, -1.000000000000000000 ) ) ;
#4059=VERTEX_POINT ( 'NONE', #24061 ) ;
#4072=PLANE ( 'NONE',  #20161 ) ;
#4073=LINE ( 'NONE', #11659, #8849 ) ;
#4078=CARTESIAN_POINT ( 'NONE',  ( 26.47460221209471598, -121.8961639463267090, 5.500000000000000000 ) ) ;
#4085=ADVANCED_FACE ( 'NONE', ( #1541 ), #1778, .F. ) ;
#4087=ORIENTED_EDGE ( 'NONE', *, *, #17802, .F. ) ;
#4092=CARTESIAN_POINT ( 'NONE',  ( -0.1219594728601508804, -118.5049662589159567, -2.500000000000000000 ) ) ;
#4095=DIRECTION ( 'NONE',  ( -0.000000000000000000, -0.000000000000000000, -1.000000000000000000 ) ) ;
#4096=CARTESIAN_POINT ( 'NONE',  ( -23.30023580412278505, -123.4057321492263384, 5.500000000000000000 ) ) ;
#4098=LINE ( 'NONE', #45944, #33426 ) ;
#4111=DIRECTION ( 'NONE',  ( 0.000000000000000000, -0.000000000000000000, 1.000000000000000000 ) ) ;
#4128=DIRECTION ( 'NONE',  ( 0.9827303690289279636, 0.1850432970638682395, -0.000000000000000000 ) ) ;
#4139=ORIENTED_EDGE ( 'NONE', *, *, #25885, .F. ) ;
#4140=CARTESIAN_POINT ( 'NONE',  ( 18.80329974962065265, -105.8248132807389084, 5.500000000000000000 ) ) ;
#4141=ORIENTED_EDGE ( 'NONE', *, *, #36477, .T. ) ;
#4151=EDGE_CURVE ( 'NONE', #31423, #46006, #21585, .T. ) ;
#4159=CARTESIAN_POINT ( 'NONE',  ( 0.000000000000000000, -120.0000000000000000, 5.500000000000000888 ) ) ;
#4163=ORIENTED_EDGE ( 'NONE', *, *, #41011, .F. ) ;
#4190=VERTEX_POINT ( 'NONE', #2037 ) ;
#4204=EDGE_CURVE ( 'NONE', #13208, #32168, #17680, .T. ) ;
#4213=PLANE ( 'NONE',  #40358 ) ;
#4217=CARTESIAN_POINT ( 'NONE',  ( -7.670864526094549163, -97.73662565058241114, -5.500000000000000000 ) ) ;
#4221=VECTOR ( 'NONE', #30298, 1000.000000000000114 ) ;
#4242=ORIENTED_EDGE ( 'NONE', *, *, #27612, .T. ) ;
#4243=ADVANCED_FACE ( 'NONE', ( #28695 ), #32594, .F. ) ;
#4255=DIRECTION ( 'NONE',  ( 0.7273375899149802093, -0.6862798483830544471, 0.000000000000000000 ) ) ;
#4261=VERTEX_POINT ( 'NONE', #40193 ) ;
#4267=CARTESIAN_POINT ( 'NONE',  ( 3.429551818649054340, -146.3199197248623875, 5.500000000000000000 ) ) ;
#4279=DIRECTION ( 'NONE',  ( -0.9827303690289279636, -0.1850432970638682117, 0.000000000000000000 ) ) ;
#4294=VECTOR ( 'NONE', #39015, 1000.000000000000000 ) ;
#4299=VECTOR ( 'NONE', #14583, 1000.000000000000000 ) ;
#4333=LINE ( 'NONE', #38097, #10249 ) ;
#4343=DIRECTION ( 'NONE',  ( 1.000000000000000000, 0.000000000000000000, -0.000000000000000000 ) ) ;
#4345=DIRECTION ( 'NONE',  ( 0.02332147558787671729, 0.9997280174009349762, -0.000000000000000000 ) ) ;
#4348=CARTESIAN_POINT ( 'NONE',  ( 5.822613034544236399, -142.8165987265839760, 5.500000000000000000 ) ) ;
#4358=ORIENTED_EDGE ( 'NONE', *, *, #3299, .F. ) ;
#4361=EDGE_LOOP ( 'NONE', ( #25135, #27732, #22578, #460 ) ) ;
#4369=VERTEX_POINT ( 'NONE', #22312 ) ;
#4385=CARTESIAN_POINT ( 'NONE',  ( 4.348517481000897078, -143.0941636721797465, -2.500000000000000000 ) ) ;
#4390=EDGE_CURVE ( 'NONE', #2942, #44487, #41164, .T. ) ;
#4393=PLANE ( 'NONE',  #34458 ) ;
#4395=DIRECTION ( 'NONE',  ( 0.000000000000000000, 1.000000000000000000, 0.000000000000000000 ) ) ;
#4398=EDGE_LOOP ( 'NONE', ( #22307, #45341, #2278, #37703 ) ) ;
#4406=VECTOR ( 'NONE', #36394, 1000.000000000000114 ) ;
#4408=FACE_OUTER_BOUND ( 'NONE', #37610, .T. ) ;
#4412=LINE ( 'NONE', #11511, #32666 ) ;
#4416=DIRECTION ( 'NONE',  ( -0.9827303690289279636, -0.1850432970638682117, 0.000000000000000000 ) ) ;
#4418=LINE ( 'NONE', #45771, #1068 ) ;
#4427=ORIENTED_EDGE ( 'NONE', *, *, #6299, .T. ) ;
#4428=ORIENTED_EDGE ( 'NONE', *, *, #42660, .T. ) ;
#4437=PLANE ( 'NONE',  #37943 ) ;
#4450=ORIENTED_EDGE ( 'NONE', *, *, #43051, .F. ) ;
#4461=DIRECTION ( 'NONE',  ( -0.000000000000000000, -0.000000000000000000, -1.000000000000000000 ) ) ;
#4487=CARTESIAN_POINT ( 'NONE',  ( 15.07208474345548055, -141.7963818439230010, -2.500000000000000000 ) ) ;
#4497=ORIENTED_EDGE ( 'NONE', *, *, #41792, .T. ) ;
#4511=PLANE ( 'NONE',  #27856 ) ;
#4526=EDGE_LOOP ( 'NONE', ( #15628, #28172, #13458, #48225 ) ) ;
#4533=DIRECTION ( 'NONE',  ( 0.7585478161175723821, 0.6516173805718057377, 0.000000000000000000 ) ) ;
#4534=ORIENTED_EDGE ( 'NONE', *, *, #38239, .F. ) ;
#4536=FACE_OUTER_BOUND ( 'NONE', #34645, .T. ) ;
#4540=DIRECTION ( 'NONE',  ( -0.6064928550163524168, -0.7950889364178789220, 0.000000000000000000 ) ) ;
#4543=MECHANICAL_DESIGN_GEOMETRIC_PRESENTATION_REPRESENTATION('',(#41345),#9328);
#4555=DIRECTION ( 'NONE',  ( -0.4279312458753000703, -0.9038112904824842087, 0.000000000000000000 ) ) ;
#4563=ADVANCED_FACE ( 'NONE', ( #741 ), #12026, .F. ) ;
#4571=CARTESIAN_POINT ( 'NONE',  ( -7.572224309238338336, -145.4393675041377492, 5.500000000000000000 ) ) ;
#4577=ORIENTED_EDGE ( 'NONE', *, *, #22021, .T. ) ;
#4587=DIRECTION ( 'NONE',  ( 0.6691306063588569053, 0.7431448254773954654, 0.000000000000000000 ) ) ;
#4596=ORIENTED_EDGE ( 'NONE', *, *, #44973, .F. ) ;
#4604=ORIENTED_EDGE ( 'NONE', *, *, #38140, .F. ) ;
#4622=CARTESIAN_POINT ( 'NONE',  ( 13.83832728059186046, -142.6495187161941089, -2.500000000000000444 ) ) ;
#4624=LINE ( 'NONE', #34232, #39081 ) ;
#4631=VECTOR ( 'NONE', #20235, 1000.000000000000000 ) ;
#4651=EDGE_CURVE ( 'NONE', #45971, #30819, #5636, .T. ) ;
#4652=ORIENTED_EDGE ( 'NONE', *, *, #25102, .F. ) ;
#4660=ORIENTED_EDGE ( 'NONE', *, *, #13597, .T. ) ;
#4664=LINE ( 'NONE', #26701, #18897 ) ;
#4673=ORIENTED_EDGE ( 'NONE', *, *, #24767, .F. ) ;
#4675=ORIENTED_EDGE ( 'NONE', *, *, #17689, .F. ) ;
#4720=DIRECTION ( 'NONE',  ( -0.9781476007338042455, -0.2079116908177664758, 0.000000000000000000 ) ) ;
#4736=EDGE_LOOP ( 'NONE', ( #6332, #5617, #16245, #14178 ) ) ;
#4743=DIRECTION ( 'NONE',  ( 1.000000000000000000, 0.000000000000000000, 0.000000000000000000 ) ) ;
#4751=FACE_OUTER_BOUND ( 'NONE', #19940, .T. ) ;
#4756=CARTESIAN_POINT ( 'NONE',  ( -25.50183398199384754, -112.6408924756582053, 5.500000000000000000 ) ) ;
#4765=ADVANCED_FACE ( 'NONE', ( #34166 ), #639, .F. ) ;
#4772=ORIENTED_EDGE ( 'NONE', *, *, #2059, .T. ) ;
#4780=EDGE_LOOP ( 'NONE', ( #43136, #47578, #17837, #18162 ) ) ;
#4789=CARTESIAN_POINT ( 'NONE',  ( 2.117611129180199558, -93.54218975225703048, 5.500000000000000000 ) ) ;
#4799=LINE ( 'NONE', #35130, #20674 ) ;
#4800=VECTOR ( 'NONE', #6678, 1000.000000000000227 ) ;
#4815=DIRECTION ( 'NONE',  ( -0.000000000000000000, -0.000000000000000000, -1.000000000000000000 ) ) ;
#4821=CARTESIAN_POINT ( 'NONE',  ( -6.112675177960399608, -145.7853679859090903, 2.500000000000000000 ) ) ;
#4822=VERTEX_POINT ( 'NONE', #45420 ) ;
#4827=LINE ( 'NONE', #19731, #28078 ) ;
#4848=PLANE ( 'NONE',  #20460 ) ;
#4863=VECTOR ( 'NONE', #45988, 1000.000000000000000 ) ;
#4870=CARTESIAN_POINT ( 'NONE',  ( -13.05994868825747446, -139.5943292883446532, -5.500000000000000000 ) ) ;
#4896=CARTESIAN_POINT ( 'NONE',  ( 12.50000000000000000, -132.5000000000000000, 2.500000000000000000 ) ) ;
#4946=VECTOR ( 'NONE', #47822, 1000.000000000000000 ) ;
#4952=AXIS2_PLACEMENT_3D ( 'NONE', #8317, #33527, #19545 ) ;
#4962=CARTESIAN_POINT ( 'NONE',  ( 24.94940289813197509, -237.3777120880564553, -5.500000000000000000 ) ) ;
#4964=VECTOR ( 'NONE', #30575, 1000.000000000000000 ) ;
#4973=AXIS2_PLACEMENT_3D ( 'NONE', #11179, #26588, #33675 ) ;
#4979=DIRECTION ( 'NONE',  ( 0.9135454576426004225, 0.4067366430758009854, 0.000000000000000000 ) ) ;
#4991=PLANE ( 'NONE',  #11503 ) ;
#4995=PLANE ( 'NONE',  #11241 ) ;
#4997=ORIENTED_EDGE ( 'NONE', *, *, #17969, .T. ) ;
#5006=VECTOR ( 'NONE', #23283, 1000.000000000000000 ) ;
#5010=ORIENTED_EDGE ( 'NONE', *, *, #46, .F. ) ;
#5030=ORIENTED_EDGE ( 'NONE', *, *, #12839, .F. ) ;
#5095=CARTESIAN_POINT ( 'NONE',  ( -4.653126046682595884, -146.1313684676804314, -2.500000000000000000 ) ) ;
#5097=ORIENTED_EDGE ( 'NONE', *, *, #15948, .T. ) ;
#5105=CARTESIAN_POINT ( 'NONE',  ( 23.11608002360578240, -124.4885236261218182, 5.500000000000000000 ) ) ;
#5112=DIRECTION ( 'NONE',  ( 0.9918136447140104561, -0.1276937514489679681, 0.000000000000000000 ) ) ;
#5116=EDGE_LOOP ( 'NONE', ( #41819, #6393, #34251, #44198 ) ) ;
#5137=DIRECTION ( 'NONE',  ( 0.3311129884571304971, 0.9435911131814395114, -0.000000000000000000 ) ) ;
#5141=ORIENTED_EDGE ( 'NONE', *, *, #43982, .F. ) ;
#5156=VERTEX_POINT ( 'NONE', #41958 ) ;
#5178=AXIS2_PLACEMENT_3D ( 'NONE', #7385, #37487, #17906 ) ;
#5183=CARTESIAN_POINT ( 'NONE',  ( 11.41210121379328335, -99.40233154247455616, 5.500000000000000000 ) ) ;
#5209=EDGE_CURVE ( 'NONE', #10969, #33189, #41463, .T. ) ;
#5216=VERTEX_POINT ( 'NONE', #40989 ) ;
#5218=ORIENTED_EDGE ( 'NONE', *, *, #38543, .F. ) ;
#5221=FACE_BOUND ( 'NONE', #20496, .T. ) ;
#5241=FACE_OUTER_BOUND ( 'NONE', #4526, .T. ) ;
#5244=PLANE ( 'NONE',  #34523 ) ;
#5271=VERTEX_POINT ( 'NONE', #11120 ) ;
#5275=ORIENTED_EDGE ( 'NONE', *, *, #25793, .F. ) ;
#5314=ADVANCED_FACE ( 'NONE', ( #45869 ), #9365, .F. ) ;
#5324=ORIENTED_EDGE ( 'NONE', *, *, #27522, .T. ) ;
#5330=EDGE_CURVE ( 'NONE', #44442, #12242, #28968, .T. ) ;
#5332=EDGE_LOOP ( 'NONE', ( #23307, #33843, #24527, #47412 ) ) ;
#5335=VERTEX_POINT ( 'NONE', #5703 ) ;
#5346=ORIENTED_EDGE ( 'NONE', *, *, #20683, .T. ) ;
#5374=VECTOR ( 'NONE', #39539, 1000.000000000000000 ) ;
#5379=CARTESIAN_POINT ( 'NONE',  ( 16.30584220631899228, -140.9432449716519784, 5.500000000000000000 ) ) ;
#5389=DIRECTION ( 'NONE',  ( 0.6862798483830533369, 0.7273375899149812085, 0.000000000000000000 ) ) ;
#5407=FACE_OUTER_BOUND ( 'NONE', #33679, .T. ) ;
#5411=DIRECTION ( 'NONE',  ( -0.5000000000000039968, 0.8660254037844363761, 0.000000000000000000 ) ) ;
#5422=CYLINDRICAL_SURFACE ( 'NONE', #16290, 35.50000000000000711 ) ;
#5425=ORIENTED_EDGE ( 'NONE', *, *, #45655, .T. ) ;
#5428=EDGE_CURVE ( 'NONE', #34042, #2158, #28458, .T. ) ;
#5433=AXIS2_PLACEMENT_3D ( 'NONE', #13009, #13239, #5411 ) ;
#5444=ORIENTED_EDGE ( 'NONE', *, *, #20210, .T. ) ;
#5465=CARTESIAN_POINT ( 'NONE',  ( 11.34017801569539685, -96.04900080221412395, -2.500000000000000000 ) ) ;
#5473=ADVANCED_FACE ( 'NONE', ( #33082 ), #36749, .F. ) ;
#5477=EDGE_CURVE ( 'NONE', #5271, #17177, #25500, .T. ) ;
#5479=STYLED_ITEM ( 'NONE', ( #40079 ), #19421 ) ;
#5486=FACE_OUTER_BOUND ( 'NONE', #22731, .T. ) ;
#5495=FACE_OUTER_BOUND ( 'NONE', #33374, .T. ) ;
#5497=LINE ( 'NONE', #8443, #19518 ) ;
#5501=VERTEX_POINT ( 'NONE', #44351 ) ;
#5549=VECTOR ( 'NONE', #13236, 1000.000000000000000 ) ;
#5552=CARTESIAN_POINT ( 'NONE',  ( -0.8815729230226008184, -93.47222532549339746, 5.500000000000000000 ) ) ;
#5559=EDGE_LOOP ( 'NONE', ( #29163, #25361 ) ) ;
#5563=VERTEX_POINT ( 'NONE', #19122 ) ;
#5588=ORIENTED_EDGE ( 'NONE', *, *, #43526, .T. ) ;
#5605=DIRECTION ( 'NONE',  ( -0.7950889364178796992, 0.6064928550163510845, 0.000000000000000000 ) ) ;
#5615=LINE ( 'NONE', #19793, #48368 ) ;
#5617=ORIENTED_EDGE ( 'NONE', *, *, #28139, .T. ) ;
#5618=AXIS2_PLACEMENT_3D ( 'NONE', #38648, #5112, #45481 ) ;
#5636=LINE ( 'NONE', #9529, #41533 ) ;
#5644=DIRECTION ( 'NONE',  ( -0.000000000000000000, -0.000000000000000000, -1.000000000000000000 ) ) ;
#5659=VECTOR ( 'NONE', #44915, 1000.000000000000000 ) ;
#5664=CARTESIAN_POINT ( 'NONE',  ( 18.80329974962065265, -105.8248132807389084, 5.500000000000000000 ) ) ;
#5666=ADVANCED_FACE ( 'NONE', ( #3468 ), #33800, .F. ) ;
#5685=CARTESIAN_POINT ( 'NONE',  ( 23.11608002360578240, -124.4885236261218182, -5.500000000000000000 ) ) ;
#5688=EDGE_CURVE ( 'NONE', #41344, #44547, #7145, .T. ) ;
#5689=DIRECTION ( 'NONE',  ( 0.000000000000000000, 0.000000000000000000, 1.000000000000000000 ) ) ;
#5703=CARTESIAN_POINT ( 'NONE',  ( 12.50000000000000000, -132.5000000000000000, -2.500000000000000000 ) ) ;
#5712=LINE ( 'NONE', #32387, #6738 ) ;
#5718=FACE_OUTER_BOUND ( 'NONE', #42996, .T. ) ;
#5725=ORIENTED_EDGE ( 'NONE', *, *, #40549, .F. ) ;
#5745=VECTOR ( 'NONE', #24036, 1000.000000000000000 ) ;
#5814=ADVANCED_FACE ( 'NONE', ( #5407 ), #31124, .F. ) ;
#5817=LINE ( 'NONE', #31529, #20367 ) ;
#5822=VERTEX_POINT ( 'NONE', #26969 ) ;
#5827=FACE_OUTER_BOUND ( 'NONE', #25533, .T. ) ;
#5846=CARTESIAN_POINT ( 'NONE',  ( 22.08297821871651934, -111.8242998470044540, 2.500000000000000000 ) ) ;
#5856=DIRECTION ( 'NONE',  ( -0.2867529058022035837, 0.9580045777625452175, 0.000000000000000000 ) ) ;
#5878=ADVANCED_FACE ( 'NONE', ( #43093 ), #43806, .F. ) ;
#5886=LINE ( 'NONE', #46989, #10593 ) ;
#5890=ORIENTED_EDGE ( 'NONE', *, *, #15873, .T. ) ;
#5906=VECTOR ( 'NONE', #47042, 1000.000000000000000 ) ;
#5908=DIRECTION ( 'NONE',  ( 0.08130631524010120681, -0.9966891607226784355, 0.000000000000000000 ) ) ;
#5913=DIRECTION ( 'NONE',  ( -0.4796670183876317051, 0.8774505977381972244, 0.000000000000000000 ) ) ;
#5936=VERTEX_POINT ( 'NONE', #32086 ) ;
#5938=EDGE_CURVE ( 'NONE', #18327, #5156, #3158, .T. ) ;
#5962=CARTESIAN_POINT ( 'NONE',  ( 19.12409105625795291, -101.5943176906707919, 5.500000000000000000 ) ) ;
#5965=AXIS2_PLACEMENT_3D ( 'NONE', #21668, #37073, #18476 ) ;
#5970=CARTESIAN_POINT ( 'NONE',  ( 19.12409105625795291, -101.5943176906707919, 5.500000000000000000 ) ) ;
#5980=EDGE_LOOP ( 'NONE', ( #38335, #35686, #23336, #34280 ) ) ;
#5988=EDGE_CURVE ( 'NONE', #21754, #36710, #26661, .T. ) ;
#6000=EDGE_CURVE ( 'NONE', #28111, #14239, #14918, .T. ) ;
#6001=CARTESIAN_POINT ( 'NONE',  ( 12.69589495141918611, -96.69089767102708777, -5.500000000000000000 ) ) ;
#6003=ORIENTED_EDGE ( 'NONE', *, *, #20846, .F. ) ;
#6013=DIRECTION ( 'NONE',  ( -0.000000000000000000, -0.000000000000000000, -1.000000000000000000 ) ) ;
#6031=CARTESIAN_POINT ( 'NONE',  ( 48.80839716909466830, -10.37454508288725208, 5.500000000000000000 ) ) ;
#6069=ORIENTED_EDGE ( 'NONE', *, *, #15539, .F. ) ;
#6077=ADVANCED_FACE ( 'NONE', ( #18587 ), #33508, .F. ) ;
#6088=LINE ( 'NONE', #21000, #15829 ) ;
#6108=AXIS2_PLACEMENT_3D ( 'NONE', #37603, #29772, #14855 ) ;
#6125=CARTESIAN_POINT ( 'NONE',  ( 30.50000000000000000, -120.0000000000000000, 2.500000000000000000 ) ) ;
#6136=DIRECTION ( 'NONE',  ( -0.1045284632676436315, -0.9945218953682742891, 0.000000000000000000 ) ) ;
#6137=DIRECTION ( 'NONE',  ( 0.7585478161175706058, 0.6516173805718080692, -0.000000000000000000 ) ) ;
#6140=FACE_OUTER_BOUND ( 'NONE', #38172, .T. ) ;
#6148=VERTEX_POINT ( 'NONE', #4622 ) ;
#6156=EDGE_CURVE ( 'NONE', #47410, #43520, #38399, .T. ) ;
#6157=LINE ( 'NONE', #13029, #35456 ) ;
#6168=ORIENTED_EDGE ( 'NONE', *, *, #15923, .F. ) ;
#6170=LINE ( 'NONE', #24771, #26612 ) ;
#6177=DIRECTION ( 'NONE',  ( -0.9827303690289279636, -0.1850432970638682117, 0.000000000000000000 ) ) ;
#6181=CARTESIAN_POINT ( 'NONE',  ( 20.85212586905262100, -130.9402397935870965, 5.500000000000000000 ) ) ;
#6194=CARTESIAN_POINT ( 'NONE',  ( 11.41210121379328335, -99.40233154247455616, 5.500000000000000000 ) ) ;
#6205=CARTESIAN_POINT ( 'NONE',  ( 32.50000000000000000, -120.0000000000000000, 2.500000000000000000 ) ) ;
#6211=EDGE_CURVE ( 'NONE', #25900, #22480, #34714, .T. ) ;
#6224=ORIENTED_EDGE ( 'NONE', *, *, #22597, .T. ) ;
#6225=VERTEX_POINT ( 'NONE', #39124 ) ;
#6245=AXIS2_PLACEMENT_3D ( 'NONE', #38977, #35535, #16694 ) ;
#6251=EDGE_CURVE ( 'NONE', #3694, #18975, #26158, .T. ) ;
#6256=DIRECTION ( 'NONE',  ( -0.000000000000000000, -0.000000000000000000, -1.000000000000000000 ) ) ;
#6261=PLANE ( 'NONE',  #37673 ) ;
#6288=VERTEX_POINT ( 'NONE', #29059 ) ;
#6299=EDGE_CURVE ( 'NONE', #28619, #21334, #9978, .T. ) ;
#6307=VECTOR ( 'NONE', #33398, 1000.000000000000227 ) ;
#6309=ORIENTED_EDGE ( 'NONE', *, *, #4204, .F. ) ;
#6310=VECTOR ( 'NONE', #12791, 1000.000000000000000 ) ;
#6322=VECTOR ( 'NONE', #45868, 1000.000000000000000 ) ;
#6326=LINE ( 'NONE', #2624, #12060 ) ;
#6332=ORIENTED_EDGE ( 'NONE', *, *, #14991, .T. ) ;
#6334=ORIENTED_EDGE ( 'NONE', *, *, #44137, .T. ) ;
#6337=ORIENTED_EDGE ( 'NONE', *, *, #6587, .F. ) ;
#6350=AXIS2_PLACEMENT_3D ( 'NONE', #25849, #36634, #25132 ) ;
#6370=VERTEX_POINT ( 'NONE', #3101 ) ;
#6371=ORIENTED_EDGE ( 'NONE', *, *, #13322, .T. ) ;
#6392=EDGE_LOOP ( 'NONE', ( #11950, #34082, #34418, #1382 ) ) ;
#6393=ORIENTED_EDGE ( 'NONE', *, *, #38974, .T. ) ;
#6411=DIRECTION ( 'NONE',  ( 0.000000000000000000, -0.000000000000000000, 1.000000000000000000 ) ) ;
#6413=DIRECTION ( 'NONE',  ( 0.5200609990132993854, 0.8541291221503274356, 0.000000000000000000 ) ) ;
#6416=EDGE_LOOP ( 'NONE', ( #6224, #35957, #42529, #14503 ) ) ;
#6425=EDGE_LOOP ( 'NONE', ( #36637, #32832, #34219, #43736 ) ) ;
#6430=ORIENTED_EDGE ( 'NONE', *, *, #41673, .T. ) ;
#6434=DIRECTION ( 'NONE',  ( -0.9997280174009349762, 0.02332147558787823691, 0.000000000000000000 ) ) ;
#6455=LINE ( 'NONE', #46854, #244 ) ;
#6458=DIRECTION ( 'NONE',  ( -0.000000000000000000, -0.000000000000000000, -1.000000000000000000 ) ) ;
#6473=AXIS2_PLACEMENT_3D ( 'NONE', #44602, #45094, #44366 ) ;
#6474=ORIENTED_EDGE ( 'NONE', *, *, #9300, .T. ) ;
#6475=PLANE ( 'NONE',  #41218 ) ;
#6484=DIRECTION ( 'NONE',  ( 0.000000000000000000, -1.000000000000000000, 0.000000000000000000 ) ) ;
#6529=CARTESIAN_POINT ( 'NONE',  ( 19.29194287201271862, -133.5026271600380880, -5.500000000000000000 ) ) ;
#6530=LINE ( 'NONE', #28801, #43060 ) ;
#6531=ORIENTED_EDGE ( 'NONE', *, *, #35711, .F. ) ;
#6549=VECTOR ( 'NONE', #3831, 1000.000000000000000 ) ;
#6552=CARTESIAN_POINT ( 'NONE',  ( -0.9515373497862389396, -96.47140937769621871, 5.500000000000000000 ) ) ;
#6568=EDGE_CURVE ( 'NONE', #18661, #41940, #15581, .T. ) ;
#6570=CARTESIAN_POINT ( 'NONE',  ( -26.29030328629083968, -123.6496510949466341, 5.500000000000000000 ) ) ;
#6577=VECTOR ( 'NONE', #20709, 1000.000000000000114 ) ;
#6587=EDGE_CURVE ( 'NONE', #19725, #28510, #17197, .T. ) ;
#6595=ORIENTED_EDGE ( 'NONE', *, *, #23769, .F. ) ;
#6598=LINE ( 'NONE', #21992, #8607 ) ;
#6619=DIRECTION ( 'NONE',  ( 0.000000000000000000, 0.000000000000000000, 1.000000000000000000 ) ) ;
#6624=AXIS2_PLACEMENT_3D ( 'NONE', #18498, #41032, #41266 ) ;
#6629=EDGE_CURVE ( 'NONE', #16756, #29948, #38106, .T. ) ;
#6634=ADVANCED_FACE ( 'NONE', ( #19473 ), #45683, .F. ) ;
#6639=LINE ( 'NONE', #7107, #12536 ) ;
#6651=EDGE_LOOP ( 'NONE', ( #39538, #36206 ) ) ;
#6656=CARTESIAN_POINT ( 'NONE',  ( -12.50000000000000000, -132.5000000000000000, 2.500000000000000000 ) ) ;
#6673=ORIENTED_EDGE ( 'NONE', *, *, #10947, .F. ) ;
#6674=EDGE_CURVE ( 'NONE', #12729, #23160, #40459, .T. ) ;
#6678=DIRECTION ( 'NONE',  ( -0.8541291221503265474, 0.5200609990133007177, 0.000000000000000000 ) ) ;
#6679=FACE_OUTER_BOUND ( 'NONE', #14679, .T. ) ;
#6715=LINE ( 'NONE', #43673, #5374 ) ;
#6732=CARTESIAN_POINT ( 'NONE',  ( 13.83832728059186046, -142.6495187161941089, 5.500000000000000000 ) ) ;
#6738=VECTOR ( 'NONE', #46836, 1000.000000000000000 ) ;
#6739=DIRECTION ( 'NONE',  ( -0.000000000000000000, -0.000000000000000000, 1.000000000000000000 ) ) ;
#6744=CARTESIAN_POINT ( 'NONE',  ( 24.95699195200416654, -110.9640411295978595, 5.500000000000000000 ) ) ;
#6773=CARTESIAN_POINT ( 'NONE',  ( -0.1915406271734583221, -121.4877204670710427, 2.500000000000000000 ) ) ;
#6781=ORIENTED_EDGE ( 'NONE', *, *, #31985, .T. ) ;
#6784=FACE_BOUND ( 'NONE', #23313, .T. ) ;
#6788=AXIS2_PLACEMENT_3D ( 'NONE', #34652, #15586, #26842 ) ;
#6792=AXIS2_PLACEMENT_3D ( 'NONE', #3107, #48157, #36881 ) ;
#6806=FACE_OUTER_BOUND ( 'NONE', #622, .T. ) ;
#6812=EDGE_CURVE ( 'NONE', #45107, #3188, #44599, .T. ) ;
#6820=ORIENTED_EDGE ( 'NONE', *, *, #11718, .T. ) ;
#6822=VECTOR ( 'NONE', #43221, 1000.000000000000114 ) ;
#6839=DIRECTION ( 'NONE',  ( -0.000000000000000000, -0.000000000000000000, -1.000000000000000000 ) ) ;
#6840=PLANE ( 'NONE',  #4005 ) ;
#6849=ADVANCED_FACE ( 'NONE', ( #41417, #23052 ), #26978, .F. ) ;
#6858=DIRECTION ( 'NONE',  ( 0.4279312458752991266, 0.9038112904824847638, 0.000000000000000000 ) ) ;
#6872=DIRECTION ( 'NONE',  ( -0.000000000000000000, -0.000000000000000000, 1.000000000000000000 ) ) ;
#6888=CARTESIAN_POINT ( 'NONE',  ( 10.05638427806949586, -98.76043467366159234, -2.500000000000000000 ) ) ;
#6889=ORIENTED_EDGE ( 'NONE', *, *, #31782, .F. ) ;
#6890=DIRECTION ( 'NONE',  ( 0.8541291221503261033, -0.5200609990133016058, 0.000000000000000000 ) ) ;
#6893=ORIENTED_EDGE ( 'NONE', *, *, #756, .F. ) ;
#6904=DIRECTION ( 'NONE',  ( 0.9918136447140100120, -0.1276937514489704939, 0.000000000000000000 ) ) ;
#6938=ORIENTED_EDGE ( 'NONE', *, *, #14821, .F. ) ;
#6939=VECTOR ( 'NONE', #24342, 1000.000000000000000 ) ;
#6947=ORIENTED_EDGE ( 'NONE', *, *, #31011, .T. ) ;
#6971=VECTOR ( 'NONE', #25644, 1000.000000000000114 ) ;
#6975=CARTESIAN_POINT ( 'NONE',  ( -18.12185313557660038, -104.9634299478706794, 5.500000000000000000 ) ) ;
#6977=VECTOR ( 'NONE', #21147, 1000.000000000000114 ) ;
#6979=LINE ( 'NONE', #32215, #6822 ) ;
#7000=LINE ( 'NONE', #25833, #29550 ) ;
#7011=LINE ( 'NONE', #28578, #27624 ) ;
#7016=DIRECTION ( 'NONE',  ( 0.9827303690289279636, 0.1850432970638681840, 0.000000000000000000 ) ) ;
#7029=VECTOR ( 'NONE', #28650, 1000.000000000000000 ) ;
#7039=AXIS2_PLACEMENT_3D ( 'NONE', #46581, #13051, #27982 ) ;
#7046=CARTESIAN_POINT ( 'NONE',  ( 48.80839716909466830, -10.37454508288725208, -5.500000000000000000 ) ) ;
#7061=ADVANCED_FACE ( 'NONE', ( #42138 ), #1269, .T. ) ;
#7071=ORIENTED_EDGE ( 'NONE', *, *, #40549, .T. ) ;
#7084=DIRECTION ( 'NONE',  ( 1.000000000000000000, 0.000000000000000000, 0.000000000000000000 ) ) ;
#7107=CARTESIAN_POINT ( 'NONE',  ( -11.59517495878806947, -96.12423995607481686, 5.500000000000000000 ) ) ;
#7108=ORIENTED_EDGE ( 'NONE', *, *, #7948, .F. ) ;
#7125=EDGE_CURVE ( 'NONE', #42528, #38227, #47011, .T. ) ;
#7138=LINE ( 'NONE', #22322, #9567 ) ;
#7143=LINE ( 'NONE', #14738, #2644 ) ;
#7145=LINE ( 'NONE', #33337, #19812 ) ;
#7156=CARTESIAN_POINT ( 'NONE',  ( -18.24502636017238899, -100.7225776329765665, 5.500000000000000000 ) ) ;
#7184=LINE ( 'NONE', #570, #10491 ) ;
#7189=ORIENTED_EDGE ( 'NONE', *, *, #25102, .T. ) ;
#7198=ORIENTED_EDGE ( 'NONE', *, *, #8538, .F. ) ;
#7203=DIRECTION ( 'NONE',  ( -0.1850432970638667129, 0.9827303690289281857, 0.000000000000000000 ) ) ;
#7207=CARTESIAN_POINT ( 'NONE',  ( -35.50000000000000711, -120.0000000000000000, 2.500000000000000000 ) ) ;
#7214=PLANE ( 'NONE',  #5965 ) ;
#7228=ORIENTED_EDGE ( 'NONE', *, *, #46135, .T. ) ;
#7230=VECTOR ( 'NONE', #12828, 1000.000000000000114 ) ;
#7232=CARTESIAN_POINT ( 'NONE',  ( 22.08297821871651934, -111.8242998470044540, 5.500000000000000000 ) ) ;
#7236=PLANE ( 'NONE',  #6624 ) ;
#7237=VERTEX_POINT ( 'NONE', #45495 ) ;
#7242=ORIENTED_EDGE ( 'NONE', *, *, #46007, .F. ) ;
#7257=LINE ( 'NONE', #4078, #33456 ) ;
#7265=CARTESIAN_POINT ( 'NONE',  ( 22.08297821871651934, -111.8242998470044540, 5.500000000000000000 ) ) ;
#7276=AXIS2_PLACEMENT_3D ( 'NONE', #7526, #18757, #3846 ) ;
#7281=ADVANCED_FACE ( 'NONE', ( #4408 ), #14689, .F. ) ;
#7293=EDGE_CURVE ( 'NONE', #9579, #6370, #18594, .T. ) ;
#7297=ORIENTED_EDGE ( 'NONE', *, *, #30792, .F. ) ;
#7309=ORIENTED_EDGE ( 'NONE', *, *, #32462, .F. ) ;
#7312=VECTOR ( 'NONE', #24686, 1000.000000000000000 ) ;
#7321=LINE ( 'NONE', #35804, #47213 ) ;
#7322=CARTESIAN_POINT ( 'NONE',  ( 12.13205353604972991, -140.1820037904669789, 5.500000000000000000 ) ) ;
#7358=ORIENTED_EDGE ( 'NONE', *, *, #39699, .T. ) ;
#7384=VECTOR ( 'NONE', #29024, 1000.000000000000114 ) ;
#7385=CARTESIAN_POINT ( 'NONE',  ( -6.880223345695647197, -142.5202692415819854, 5.500000000000000000 ) ) ;
#7387=VECTOR ( 'NONE', #39753, 1000.000000000000114 ) ;
#7401=FACE_OUTER_BOUND ( 'NONE', #4361, .T. ) ;
#7405=ADVANCED_FACE ( 'NONE', ( #1204 ), #34969, .F. ) ;
#7410=EDGE_CURVE ( 'NONE', #35739, #35538, #12704, .T. ) ;
#7427=ORIENTED_EDGE ( 'NONE', *, *, #43526, .F. ) ;
#7431=DIRECTION ( 'NONE',  ( -0.1276937514489679404, -0.9918136447140103451, 0.000000000000000000 ) ) ;
#7435=ORIENTED_EDGE ( 'NONE', *, *, #35651, .T. ) ;
#7442=CARTESIAN_POINT ( 'NONE',  ( 35.50000000000000711, -120.0000000000000000, 2.500000000000000000 ) ) ;
#7446=ORIENTED_EDGE ( 'NONE', *, *, #41082, .T. ) ;
#7469=VECTOR ( 'NONE', #43388, 1000.000000000000000 ) ;
#7474=AXIS2_PLACEMENT_3D ( 'NONE', #7924, #44653, #15296 ) ;
#7475=DIRECTION ( 'NONE',  ( -0.000000000000000000, -0.000000000000000000, -1.000000000000000000 ) ) ;
#7479=ORIENTED_EDGE ( 'NONE', *, *, #23360, .F. ) ;
#7491=DIRECTION ( 'NONE',  ( 0.000000000000000000, 0.000000000000000000, 1.000000000000000000 ) ) ;
#7496=ORIENTED_EDGE ( 'NONE', *, *, #26251, .F. ) ;
#7511=LINE ( 'NONE', #37360, #6549 ) ;
#7519=ORIENTED_EDGE ( 'NONE', *, *, #17344, .T. ) ;
#7524=AXIS2_PLACEMENT_3D ( 'NONE', #45092, #41912, #15240 ) ;
#7526=CARTESIAN_POINT ( 'NONE',  ( 14.59956846177685996, -138.4757300459248484, 5.500000000000000000 ) ) ;
#7528=EDGE_CURVE ( 'NONE', #21034, #21021, #24437, .T. ) ;
#7532=DIRECTION ( 'NONE',  ( 0.4279312458753000703, 0.9038112904824842087, 0.000000000000000000 ) ) ;
#7544=DIRECTION ( 'NONE',  ( 0.5687579148473765889, -0.8225049752423776450, 0.000000000000000000 ) ) ;
#7552=AXIS2_PLACEMENT_3D ( 'NONE', #32821, #16947, #10313 ) ;
#7562=CARTESIAN_POINT ( 'NONE',  ( 8.700667342345820288, -98.11853780484867116, -5.500000000000000000 ) ) ;
#7566=FACE_OUTER_BOUND ( 'NONE', #16870, .T. ) ;
#7578=EDGE_CURVE ( 'NONE', #37298, #3370, #47658, .T. ) ;
#7580=CARTESIAN_POINT ( 'NONE',  ( 22.51310757741980240, -113.2613067136482101, -2.500000000000000000 ) ) ;
#7581=DIRECTION ( 'NONE',  ( 0.3311129884571281101, 0.9435911131814402886, -0.000000000000000000 ) ) ;
#7593=DIRECTION ( 'NONE',  ( 1.000000000000000000, 0.000000000000000000, 0.000000000000000000 ) ) ;
#7594=FACE_OUTER_BOUND ( 'NONE', #23487, .T. ) ;
#7610=ORIENTED_EDGE ( 'NONE', *, *, #36844, .T. ) ;
#7624=DIRECTION ( 'NONE',  ( -0.000000000000000000, -0.000000000000000000, -1.000000000000000000 ) ) ;
#7637=LINE ( 'NONE', #25507, #36428 ) ;
#7638=CARTESIAN_POINT ( 'NONE',  ( 13.83832728059186046, -142.6495187161941089, 5.500000000000000000 ) ) ;
#7661=VECTOR ( 'NONE', #14623, 1000.000000000000000 ) ;
#7662=EDGE_CURVE ( 'NONE', #36733, #44017, #39040, .T. ) ;
#7664=PLANE ( 'NONE',  #28895 ) ;
#7666=ORIENTED_EDGE ( 'NONE', *, *, #16209, .T. ) ;
#7679=VERTEX_POINT ( 'NONE', #28033 ) ;
#7698=EDGE_CURVE ( 'NONE', #41154, #41259, #24343, .T. ) ;
#7709=ORIENTED_EDGE ( 'NONE', *, *, #14574, .T. ) ;
#7713=VERTEX_POINT ( 'NONE', #20676 ) ;
#7719=FACE_OUTER_BOUND ( 'NONE', #33668, .T. ) ;
#7740=LINE ( 'NONE', #19240, #43308 ) ;
#7757=DIRECTION ( 'NONE',  ( 0.6862798483830533369, 0.7273375899149812085, -0.000000000000000000 ) ) ;
#7762=DIRECTION ( 'NONE',  ( -0.9997280174009349762, 0.02332147558787823691, 0.000000000000000000 ) ) ;
#7773=VECTOR ( 'NONE', #30435, 1000.000000000000227 ) ;
#7779=EDGE_CURVE ( 'NONE', #6370, #33987, #32187, .T. ) ;
#7782=EDGE_CURVE ( 'NONE', #36901, #14848, #33519, .T. ) ;
#7783=CARTESIAN_POINT ( 'NONE',  ( -22.67106064244953245, -113.6342314410295842, 5.500000000000000000 ) ) ;
#7813=DIRECTION ( 'NONE',  ( -0.000000000000000000, -0.000000000000000000, -1.000000000000000000 ) ) ;
#7815=DIRECTION ( 'NONE',  ( 0.6516173805718058487, -0.7585478161175724932, 0.000000000000000000 ) ) ;
#7828=EDGE_CURVE ( 'NONE', #35093, #45508, #3263, .T. ) ;
#7853=CARTESIAN_POINT ( 'NONE',  ( -19.90058851926621131, -132.5883508287165853, 2.500000000000000000 ) ) ;
#7858=VERTEX_POINT ( 'NONE', #22600 ) ;
#7866=DIRECTION ( 'NONE',  ( -0.000000000000000000, -0.000000000000000000, -1.000000000000000000 ) ) ;
#7890=EDGE_CURVE ( 'NONE', #29100, #41379, #18911, .T. ) ;
#7910=EDGE_LOOP ( 'NONE', ( #35360, #38006, #46552, #48130 ) ) ;
#7924=CARTESIAN_POINT ( 'NONE',  ( -17.26469406256017791, -140.1601175325492648, 5.500000000000000000 ) ) ;
#7948=EDGE_CURVE ( 'NONE', #30446, #23907, #15504, .T. ) ;
#7969=PLANE ( 'NONE',  #4973 ) ;
#7988=DIRECTION ( 'NONE',  ( -0.08130631524010122069, 0.9966891607226784355, 0.000000000000000000 ) ) ;
#7994=AXIS2_PLACEMENT_3D ( 'NONE', #40089, #44718, #43996 ) ;
#8017=LINE ( 'NONE', #446, #26634 ) ;
#8057=DIRECTION ( 'NONE',  ( 0.9966891607226785466, 0.08130631524010119293, -0.000000000000000000 ) ) ;
#8058=ADVANCED_FACE ( 'NONE', ( #37891 ), #15140, .F. ) ;
#8082=VECTOR ( 'NONE', #13125, 1000.000000000000114 ) ;
#8090=CARTESIAN_POINT ( 'NONE',  ( 26.47460221209471953, -121.8961639463267090, -2.500000000000000000 ) ) ;
#8096=LINE ( 'NONE', #46036, #27396 ) ;
#8104=ORIENTED_EDGE ( 'NONE', *, *, #21080, .F. ) ;
#8112=LINE ( 'NONE', #37985, #22347 ) ;
#8120=CARTESIAN_POINT ( 'NONE',  ( -12.50000000000000000, -132.5000000000000000, -2.500000000000000000 ) ) ;
#8139=VERTEX_POINT ( 'NONE', #43250 ) ;
#8146=DIRECTION ( 'NONE',  ( 0.08130631524010120681, -0.9966891607226784355, 0.000000000000000000 ) ) ;
#8168=FACE_OUTER_BOUND ( 'NONE', #17714, .T. ) ;
#8171=LINE ( 'NONE', #30685, #23770 ) ;
#8182=DIRECTION ( 'NONE',  ( 0.8225049752423786442, 0.5687579148473752566, -0.000000000000000000 ) ) ;
#8189=EDGE_CURVE ( 'NONE', #25651, #35339, #31282, .T. ) ;
#8201=CARTESIAN_POINT ( 'NONE',  ( 2.117611129180199558, -93.54218975225703048, -5.500000000000000000 ) ) ;
#8225=DIRECTION ( 'NONE',  ( -0.8090169943749504489, 0.5877852522924689183, 0.000000000000000000 ) ) ;
#8230=DIRECTION ( 'NONE',  ( -0.8225049752423776450, -0.5687579148473765889, 0.000000000000000000 ) ) ;
#8234=AXIS2_PLACEMENT_3D ( 'NONE', #46627, #2081, #32421 ) ;
#8235=ORIENTED_EDGE ( 'NONE', *, *, #47916, .T. ) ;
#8240=FACE_OUTER_BOUND ( 'NONE', #3198, .T. ) ;
#8243=EDGE_CURVE ( 'NONE', #46631, #16756, #43013, .T. ) ;
#8247=LINE ( 'NONE', #15366, #1355 ) ;
#8249=VECTOR ( 'NONE', #14510, 1000.000000000000227 ) ;
#8250=FACE_OUTER_BOUND ( 'NONE', #16828, .T. ) ;
#8251=DIRECTION ( 'NONE',  ( -0.000000000000000000, -0.000000000000000000, -1.000000000000000000 ) ) ;
#8262=PLANE ( 'NONE',  #17135 ) ;
#8267=EDGE_LOOP ( 'NONE', ( #14359, #39111, #31828, #38799 ) ) ;
#8269=ORIENTED_EDGE ( 'NONE', *, *, #46189, .T. ) ;
#8289=VECTOR ( 'NONE', #45817, 1000.000000000000000 ) ;
#8302=EDGE_CURVE ( 'NONE', #34545, #42101, #10439, .T. ) ;
#8313=ORIENTED_EDGE ( 'NONE', *, *, #11995, .F. ) ;
#8317=CARTESIAN_POINT ( 'NONE',  ( 0.000000000000000000, -120.0000000000000000, 2.500000000000000000 ) ) ;
#8324=ORIENTED_EDGE ( 'NONE', *, *, #12136, .F. ) ;
#8327=DIRECTION ( 'NONE',  ( 0.000000000000000000, -1.000000000000000000, 0.000000000000000000 ) ) ;
#8332=CARTESIAN_POINT ( 'NONE',  ( -24.50849501662245800, -109.8101191361138831, 5.500000000000000000 ) ) ;
#8334=EDGE_CURVE ( 'NONE', #22480, #41344, #7000, .T. ) ;
#8337=EDGE_CURVE ( 'NONE', #14239, #10647, #14610, .T. ) ;
#8343=ORIENTED_EDGE ( 'NONE', *, *, #14574, .F. ) ;
#8351=LINE ( 'NONE', #15692, #5006 ) ;
#8353=CARTESIAN_POINT ( 'NONE',  ( 8.700667342345820288, -98.11853780484867116, 5.500000000000000000 ) ) ;
#8358=EDGE_CURVE ( 'NONE', #23160, #3234, #33195, .T. ) ;
#8364=LINE ( 'NONE', #18415, #42814 ) ;
#8377=VERTEX_POINT ( 'NONE', #2360 ) ;
#8404=EDGE_CURVE ( 'NONE', #24649, #27608, #47630, .T. ) ;
#8406=VECTOR ( 'NONE', #7988, 1000.000000000000114 ) ;
#8414=ADVANCED_FACE ( 'NONE', ( #11422 ), #15334, .F. ) ;
#8415=DIRECTION ( 'NONE',  ( -0.000000000000000000, -0.000000000000000000, -1.000000000000000000 ) ) ;
#8441=LINE ( 'NONE', #19440, #19870 ) ;
#8443=CARTESIAN_POINT ( 'NONE',  ( -1.499592026101402853, -119.9650177866181764, 2.500000000000000000 ) ) ;
#8445=ORIENTED_EDGE ( 'NONE', *, *, #14700, .T. ) ;
#8447=ORIENTED_EDGE ( 'NONE', *, *, #25689, .T. ) ;
#8455=ORIENTED_EDGE ( 'NONE', *, *, #28139, .F. ) ;
#8456=FACE_OUTER_BOUND ( 'NONE', #29471, .T. ) ;
#8467=LINE ( 'NONE', #31243, #43874 ) ;
#8470=DIRECTION ( 'NONE',  ( 0.000000000000000000, 0.000000000000000000, 1.000000000000000000 ) ) ;
#8475=DIRECTION ( 'NONE',  ( -0.000000000000000000, -0.000000000000000000, -1.000000000000000000 ) ) ;
#8476=FACE_OUTER_BOUND ( 'NONE', #36984, .T. ) ;
#8479=CARTESIAN_POINT ( 'NONE',  ( -19.27444613274700913, -101.8135840178490668, 2.500000000000000000 ) ) ;
#8481=ORIENTED_EDGE ( 'NONE', *, *, #47504, .F. ) ;
#8485=ORIENTED_EDGE ( 'NONE', *, *, #33686, .T. ) ;
#8515=VERTEX_POINT ( 'NONE', #44939 ) ;
#8525=CARTESIAN_POINT ( 'NONE',  ( 17.82587367876289974, -104.6869915565625320, 2.500000000000000000 ) ) ;
#8538=EDGE_CURVE ( 'NONE', #21261, #20465, #29757, .T. ) ;
#8553=EDGE_CURVE ( 'NONE', #22152, #18327, #34621, .T. ) ;
#8597=CARTESIAN_POINT ( 'NONE',  ( -3.961125083139900749, -143.2122702051246677, 5.500000000000000000 ) ) ;
#8598=AXIS2_PLACEMENT_3D ( 'NONE', #37036, #65, #15017 ) ;
#8602=EDGE_CURVE ( 'NONE', #1613, #5563, #16771, .T. ) ;
#8607=VECTOR ( 'NONE', #6839, 1000.000000000000000 ) ;
#8616=LINE ( 'NONE', #792, #27001 ) ;
#8638=LINE ( 'NONE', #12103, #25285 ) ;
#8648=LINE ( 'NONE', #37800, #26858 ) ;
#8654=PLANE ( 'NONE',  #34680 ) ;
#8664=VECTOR ( 'NONE', #11703, 1000.000000000000114 ) ;
#8674=ORIENTED_EDGE ( 'NONE', *, *, #11932, .T. ) ;
#8693=CARTESIAN_POINT ( 'NONE',  ( 20.07203437053270179, -132.2214334768125354, 2.500000000000000000 ) ) ;
#8729=ORIENTED_EDGE ( 'NONE', *, *, #15155, .F. ) ;
#8757=ORIENTED_EDGE ( 'NONE', *, *, #8776, .T. ) ;
#8766=CARTESIAN_POINT ( 'NONE',  ( -20.62008904684763166, -131.2721749321093512, -2.500000000000000000 ) ) ;
#8767=CARTESIAN_POINT ( 'NONE',  ( 14.59956846177685996, -138.4757300459248484, 5.500000000000000000 ) ) ;
#8776=EDGE_CURVE ( 'NONE', #46691, #36404, #6715, .T. ) ;
#8780=EDGE_CURVE ( 'NONE', #35445, #36858, #10136, .T. ) ;
#8781=ORIENTED_EDGE ( 'NONE', *, *, #23769, .T. ) ;
#8800=ORIENTED_EDGE ( 'NONE', *, *, #45976, .F. ) ;
#8815=ORIENTED_EDGE ( 'NONE', *, *, #44001, .T. ) ;
#8822=LINE ( 'NONE', #41900, #18037 ) ;
#8830=CARTESIAN_POINT ( 'NONE',  ( -0.7195005275814509993, -118.6838241033926948, -2.500000000000000000 ) ) ;
#8839=ORIENTED_EDGE ( 'NONE', *, *, #12073, .F. ) ;
#8849=VECTOR ( 'NONE', #4555, 1000.000000000000114 ) ;
#8853=ORIENTED_EDGE ( 'NONE', *, *, #42836, .F. ) ;
#8860=AXIS2_PLACEMENT_3D ( 'NONE', #42091, #3915, #18830 ) ;
#8864=CARTESIAN_POINT ( 'NONE',  ( -23.30023580412278505, -123.4057321492263384, 5.500000000000000000 ) ) ;
#8868=DIRECTION ( 'NONE',  ( -0.7950889364178796992, 0.6064928550163510845, 0.000000000000000000 ) ) ;
#8883=VECTOR ( 'NONE', #41544, 1000.000000000000114 ) ;
#8902=DIRECTION ( 'NONE',  ( -0.5687579148473752566, 0.8225049752423786442, 0.000000000000000000 ) ) ;
#8907=CARTESIAN_POINT ( 'NONE',  ( 26.09152095774781799, -124.8716048804687375, 5.500000000000000000 ) ) ;
#8912=VECTOR ( 'NONE', #42698, 1000.000000000000114 ) ;
#8923=CARTESIAN_POINT ( 'NONE',  ( -26.29030328629083968, -123.6496510949466341, 5.500000000000000000 ) ) ;
#8937=ORIENTED_EDGE ( 'NONE', *, *, #11995, .T. ) ;
#8962=EDGE_CURVE ( 'NONE', #31729, #35538, #7184, .T. ) ;
#8963=EDGE_CURVE ( 'NONE', #44017, #25896, #37044, .T. ) ;
#8965=DIRECTION ( 'NONE',  ( -0.000000000000000000, -0.000000000000000000, -1.000000000000000000 ) ) ;
#8974=ORIENTED_EDGE ( 'NONE', *, *, #9761, .F. ) ;
#8987=VECTOR ( 'NONE', #14303, 1000.000000000000000 ) ;
#8990=ORIENTED_EDGE ( 'NONE', *, *, #8334, .T. ) ;
#8994=ORIENTED_EDGE ( 'NONE', *, *, #42066, .F. ) ;
#9019=ORIENTED_EDGE ( 'NONE', *, *, #16869, .T. ) ;
#9037=EDGE_CURVE ( 'NONE', #43974, #27838, #15987, .T. ) ;
#9044=DIRECTION ( 'NONE',  ( -0.9435911131814402886, 0.3311129884571281101, 0.000000000000000000 ) ) ;
#9062=CARTESIAN_POINT ( 'NONE',  ( -7.572224309238338336, -145.4393675041377492, -2.500000000000000444 ) ) ;
#9095=CARTESIAN_POINT ( 'NONE',  ( 26.09152095774781444, -124.8716048804687375, 2.500000000000000000 ) ) ;
#9100=VECTOR ( 'NONE', #7813, 1000.000000000000000 ) ;
#9108=AXIS2_PLACEMENT_3D ( 'NONE', #28400, #47250, #6136 ) ;
#9120=VECTOR ( 'NONE', #4095, 1000.000000000000000 ) ;
#9121=FACE_BOUND ( 'NONE', #40734, .T. ) ;
#9150=LINE ( 'NONE', #20158, #7230 ) ;
#9154=VECTOR ( 'NONE', #40684, 1000.000000000000114 ) ;
#9158=ORIENTED_EDGE ( 'NONE', *, *, #27356, .F. ) ;
#9167=CARTESIAN_POINT ( 'NONE',  ( -14.87942725330654348, -141.9795960975983178, 5.500000000000000000 ) ) ;
#9174=EDGE_CURVE ( 'NONE', #18614, #21261, #47743, .T. ) ;
#9176=EDGE_CURVE ( 'NONE', #24549, #10969, #17895, .T. ) ;
#9192=LINE ( 'NONE', #15813, #19772 ) ;
#9193=CARTESIAN_POINT ( 'NONE',  ( -0.9515373497862389396, -96.47140937769621871, -5.500000000000000000 ) ) ;
#9199=PLANE ( 'NONE',  #25408 ) ;
#9209=VERTEX_POINT ( 'NONE', #6656 ) ;
#9213=ORIENTED_EDGE ( 'NONE', *, *, #5330, .T. ) ;
#9230=EDGE_CURVE ( 'NONE', #39825, #10102, #28199, .T. ) ;
#9256=EDGE_LOOP ( 'NONE', ( #24706, #3432, #31118, #34132 ) ) ;
#9259=DIRECTION ( 'NONE',  ( -0.7950889364178796992, 0.6064928550163511956, 0.000000000000000000 ) ) ;
#9296=ORIENTED_EDGE ( 'NONE', *, *, #7890, .F. ) ;
#9300=EDGE_CURVE ( 'NONE', #2423, #45055, #15214, .T. ) ;
#9302=DIRECTION ( 'NONE',  ( -0.000000000000000000, -0.000000000000000000, -1.000000000000000000 ) ) ;
#9325=DIRECTION ( 'NONE',  ( 1.000000000000000000, 0.000000000000000000, 0.000000000000000000 ) ) ;
#9328=( GEOMETRIC_REPRESENTATION_CONTEXT ( 3 ) GLOBAL_UNCERTAINTY_ASSIGNED_CONTEXT ( ( #36944 ) ) GLOBAL_UNIT_ASSIGNED_CONTEXT ( ( #46490, #31323, #35213 ) ) REPRESENTATION_CONTEXT ( 'NONE', 'WORKASPACE' ) );
#9329=ORIENTED_EDGE ( 'NONE', *, *, #27901, .T. ) ;
#9365=PLANE ( 'NONE',  #9442 ) ;
#9432=DIRECTION ( 'NONE',  ( -0.9730327541852491491, 0.2306669878475648139, 0.000000000000000000 ) ) ;
#9442=AXIS2_PLACEMENT_3D ( 'NONE', #34834, #39000, #12812 ) ;
#9467=VECTOR ( 'NONE', #23762, 1000.000000000000000 ) ;
#9478=CARTESIAN_POINT ( 'NONE',  ( 12.69589495141918611, -96.69089767102708777, -2.500000000000000444 ) ) ;
#9489=AXIS2_PLACEMENT_3D ( 'NONE', #4896, #31106, #12495 ) ;
#9492=DIRECTION ( 'NONE',  ( 0.9435911131814402886, -0.3311129884571281101, 0.000000000000000000 ) ) ;
#9507=VECTOR ( 'NONE', #37295, 1000.000000000000114 ) ;
#9523=CARTESIAN_POINT ( 'NONE',  ( 13.83832728059186046, -142.6495187161941089, 2.500000000000000000 ) ) ;
#9525=PLANE ( 'NONE',  #3228 ) ;
#9529=CARTESIAN_POINT ( 'NONE',  ( -26.41226275915097332, -122.1546173538626761, -2.500000000000000000 ) ) ;
#9543=FACE_OUTER_BOUND ( 'NONE', #18309, .T. ) ;
#9554=CARTESIAN_POINT ( 'NONE',  ( 16.84844760790522855, -103.5491698323862124, 5.500000000000000000 ) ) ;
#9567=VECTOR ( 'NONE', #40444, 1000.000000000000000 ) ;
#9570=EDGE_LOOP ( 'NONE', ( #44078, #11726, #14167, #23241 ) ) ;
#9573=ORIENTED_EDGE ( 'NONE', *, *, #4151, .F. ) ;
#9579=VERTEX_POINT ( 'NONE', #46706 ) ;
#9584=DIRECTION ( 'NONE',  ( -0.1850432970638682395, 0.9827303690289280746, 0.000000000000000000 ) ) ;
#9622=LINE ( 'NONE', #9878, #40087 ) ;
#9669=CARTESIAN_POINT ( 'NONE',  ( -8.826826895187510402, -94.96827758698185562, 5.500000000000000000 ) ) ;
#9670=CARTESIAN_POINT ( 'NONE',  ( -0.9515373497862389396, -96.47140937769621871, 5.500000000000000000 ) ) ;
#9695=VECTOR ( 'NONE', #24487, 1000.000000000000114 ) ;
#9698=ORIENTED_EDGE ( 'NONE', *, *, #32214, .F. ) ;
#9703=EDGE_CURVE ( 'NONE', #28619, #17612, #17546, .T. ) ;
#9730=EDGE_LOOP ( 'NONE', ( #35885, #32627, #9213, #46242 ) ) ;
#9734=ORIENTED_EDGE ( 'NONE', *, *, #10339, .T. ) ;
#9737=CARTESIAN_POINT ( 'NONE',  ( 12.50000000000000000, -132.5000000000000000, 2.500000000000000000 ) ) ;
#9746=ORIENTED_EDGE ( 'NONE', *, *, #10263, .T. ) ;
#9748=CARTESIAN_POINT ( 'NONE',  ( -7.572224309238338336, -145.4393675041377492, -5.500000000000000000 ) ) ;
#9761=EDGE_CURVE ( 'NONE', #27123, #5156, #34634, .T. ) ;
#9763=VECTOR ( 'NONE', #11740, 1000.000000000000000 ) ;
#9770=EDGE_CURVE ( 'NONE', #46921, #28791, #11436, .T. ) ;
#9784=ORIENTED_EDGE ( 'NONE', *, *, #22828, .F. ) ;
#9787=DIRECTION ( 'NONE',  ( -0.5200609990132993854, -0.8541291221503275466, 0.000000000000000000 ) ) ;
#9790=FACE_OUTER_BOUND ( 'NONE', #40298, .T. ) ;
#9793=VERTEX_POINT ( 'NONE', #864 ) ;
#9837=CARTESIAN_POINT ( 'NONE',  ( 0.000000000000000000, -120.0000000000000000, 2.500000000000000000 ) ) ;
#9840=CARTESIAN_POINT ( 'NONE',  ( 0.7195005275814480017, -121.3161758966073052, 2.500000000000000000 ) ) ;
#9862=ADVANCED_FACE ( 'NONE', ( #44700 ), #7969, .F. ) ;
#9878=CARTESIAN_POINT ( 'NONE',  ( 13.36581099891334645, -139.3288669181958710, -2.500000000000000000 ) ) ;
#9881=ORIENTED_EDGE ( 'NONE', *, *, #4390, .T. ) ;
#9884=EDGE_CURVE ( 'NONE', #8515, #10011, #7740, .T. ) ;
#9889=EDGE_CURVE ( 'NONE', #26989, #1613, #7511, .T. ) ;
#9892=AXIS2_PLACEMENT_3D ( 'NONE', #165, #15833, #7532 ) ;
#9898=ORIENTED_EDGE ( 'NONE', *, *, #6568, .T. ) ;
#9902=VERTEX_POINT ( 'NONE', #42482 ) ;
#9931=CARTESIAN_POINT ( 'NONE',  ( -30.50000000000000000, -120.0000000000000000, 2.500000000000000000 ) ) ;
#9956=ORIENTED_EDGE ( 'NONE', *, *, #21080, .T. ) ;
#9958=DIRECTION ( 'NONE',  ( 0.8541291221503265474, -0.5200609990133007177, 0.000000000000000000 ) ) ;
#9961=FACE_OUTER_BOUND ( 'NONE', #41153, .T. ) ;
#9978=LINE ( 'NONE', #35695, #20666 ) ;
#9982=ORIENTED_EDGE ( 'NONE', *, *, #31782, .T. ) ;
#9995=EDGE_CURVE ( 'NONE', #2795, #12057, #46647, .T. ) ;
#10006=ORIENTED_EDGE ( 'NONE', *, *, #8963, .T. ) ;
#10011=VERTEX_POINT ( 'NONE', #16062 ) ;
#10016=LINE ( 'NONE', #44025, #47058 ) ;
#10029=LINE ( 'NONE', #43571, #33049 ) ;
#10031=ORIENTED_EDGE ( 'NONE', *, *, #18712, .F. ) ;
#10062=( GEOMETRIC_REPRESENTATION_CONTEXT ( 3 ) GLOBAL_UNCERTAINTY_ASSIGNED_CONTEXT ( ( #10542 ) ) GLOBAL_UNIT_ASSIGNED_CONTEXT ( ( #22993, #26916, #42085 ) ) REPRESENTATION_CONTEXT ( 'NONE', 'WORKASPACE' ) );
#10064=CARTESIAN_POINT ( 'NONE',  ( 16.30584220631899228, -140.9432449716519784, -2.500000000000000000 ) ) ;
#10073=ORIENTED_EDGE ( 'NONE', *, *, #43051, .T. ) ;
#10091=VERTEX_POINT ( 'NONE', #17961 ) ;
#10096=CARTESIAN_POINT ( 'NONE',  ( 21.85433023846372436, -135.0628101570779620, 2.500000000000000000 ) ) ;
#10102=VERTEX_POINT ( 'NONE', #43920 ) ;
#10105=CARTESIAN_POINT ( 'NONE',  ( 19.12409105625796357, -101.5943176906707919, -2.500000000000000000 ) ) ;
#10136=LINE ( 'NONE', #36328, #32721 ) ;
#10175=AXIS2_PLACEMENT_3D ( 'NONE', #39940, #43840, #32359 ) ;
#10197=CARTESIAN_POINT ( 'NONE',  ( -11.59517495878806947, -96.12423995607481686, 5.500000000000000000 ) ) ;
#10204=DIRECTION ( 'NONE',  ( 0.6862798483830534479, 0.7273375899149810975, 0.000000000000000000 ) ) ;
#10215=ADVANCED_FACE ( 'NONE', ( #8168 ), #38036, .F. ) ;
#10224=CARTESIAN_POINT ( 'NONE',  ( 26.47460221209471598, -121.8961639463267090, 5.500000000000000000 ) ) ;
#10232=EDGE_LOOP ( 'NONE', ( #22997, #18685, #18658, #32995 ) ) ;
#10239=AXIS2_PLACEMENT_3D ( 'NONE', #34390, #15347, #8225 ) ;
#10249=VECTOR ( 'NONE', #27085, 1000.000000000000227 ) ;
#10263=EDGE_CURVE ( 'NONE', #44807, #46921, #4019, .T. ) ;
#10282=DIRECTION ( 'NONE',  ( 0.3853207896976547087, -0.9227826878668540234, 0.000000000000000000 ) ) ;
#10283=LINE ( 'NONE', #44537, #20663 ) ;
#10301=VERTEX_POINT ( 'NONE', #12100 ) ;
#10313=DIRECTION ( 'NONE',  ( 1.000000000000000000, 0.000000000000000000, 0.000000000000000000 ) ) ;
#10317=CARTESIAN_POINT ( 'NONE',  ( 13.83832728059186046, -142.6495187161941089, -5.500000000000000000 ) ) ;
#10320=DIRECTION ( 'NONE',  ( -0.4796670183876294291, 0.8774505977381983346, 0.000000000000000000 ) ) ;
#10339=EDGE_CURVE ( 'NONE', #22480, #3571, #33393, .T. ) ;
#10380=VECTOR ( 'NONE', #11549, 1000.000000000000114 ) ;
#10391=ORIENTED_EDGE ( 'NONE', *, *, #39800, .T. ) ;
#10394=EDGE_CURVE ( 'NONE', #3684, #46691, #19898, .T. ) ;
#10404=CARTESIAN_POINT ( 'NONE',  ( -114.1267819554185365, -82.91796067500661138, 5.500000000000000000 ) ) ;
#10411=PLANE ( 'NONE',  #44961 ) ;
#10413=LINE ( 'NONE', #11144, #5659 ) ;
#10430=PLANE ( 'NONE',  #10540 ) ;
#10439=LINE ( 'NONE', #40540, #27222 ) ;
#10441=PLANE ( 'NONE',  #18058 ) ;
#10443=ORIENTED_EDGE ( 'NONE', *, *, #6674, .T. ) ;
#10444=LINE ( 'NONE', #25605, #3647 ) ;
#10445=ORIENTED_EDGE ( 'NONE', *, *, #9703, .T. ) ;
#10456=FACE_OUTER_BOUND ( 'NONE', #254, .T. ) ;
#10458=ORIENTED_EDGE ( 'NONE', *, *, #14991, .F. ) ;
#10461=EDGE_LOOP ( 'NONE', ( #44314, #4163, #13938, #26516 ) ) ;
#10469=EDGE_CURVE ( 'NONE', #29809, #21999, #23334, .T. ) ;
#10487=VECTOR ( 'NONE', #3548, 1000.000000000000114 ) ;
#10491=VECTOR ( 'NONE', #10865, 1000.000000000000000 ) ;
#10533=DIRECTION ( 'NONE',  ( -0.000000000000000000, -0.000000000000000000, 1.000000000000000000 ) ) ;
#10540=AXIS2_PLACEMENT_3D ( 'NONE', #48352, #25348, #14833 ) ;
#10542=UNCERTAINTY_MEASURE_WITH_UNIT (LENGTH_MEASURE( 1.000000000000000082E-05 ), #22993, 'distance_accuracy_value', 'NONE');
#10543=VECTOR ( 'NONE', #8475, 1000.000000000000000 ) ;
#10552=EDGE_CURVE ( 'NONE', #40846, #5216, #43629, .T. ) ;
#10576=LINE ( 'NONE', #25004, #7469 ) ;
#10593=VECTOR ( 'NONE', #12987, 1000.000000000000114 ) ;
#10602=AXIS2_PLACEMENT_3D ( 'NONE', #46233, #23969, #1451 ) ;
#10611=ORIENTED_EDGE ( 'NONE', *, *, #14550, .F. ) ;
#10612=CARTESIAN_POINT ( 'NONE',  ( -26.53422223201112828, -120.6595836127786043, -2.500000000000000444 ) ) ;
#10620=ORIENTED_EDGE ( 'NONE', *, *, #7782, .T. ) ;
#10631=ADVANCED_FACE ( 'NONE', ( #33336 ), #41643, .F. ) ;
#10647=VERTEX_POINT ( 'NONE', #23040 ) ;
#10648=PLANE ( 'NONE',  #14379 ) ;
#10701=DIRECTION ( 'NONE',  ( -0.9580045777625459946, -0.2867529058022011412, 0.000000000000000000 ) ) ;
#10722=APPLICATION_CONTEXT ( 'automotive_design' ) ;
#10756=DIRECTION ( 'NONE',  ( 0.9966891607226785466, 0.08130631524009969413, 0.000000000000000000 ) ) ;
#10760=FACE_OUTER_BOUND ( 'NONE', #35664, .T. ) ;
#10762=EDGE_LOOP ( 'NONE', ( #20425, #26920, #12967, #47423 ) ) ;
#10770=LINE ( 'NONE', #44053, #3683 ) ;
#10788=ORIENTED_EDGE ( 'NONE', *, *, #28069, .F. ) ;
#10800=LINE ( 'NONE', #14473, #31336 ) ;
#10803=LINE ( 'NONE', #25708, #46252 ) ;
#10827=DIRECTION ( 'NONE',  ( -0.9038112904824853189, 0.4279312458752977943, 0.000000000000000000 ) ) ;
#10865=DIRECTION ( 'NONE',  ( -0.000000000000000000, -0.000000000000000000, -1.000000000000000000 ) ) ;
#10872=ORIENTED_EDGE ( 'NONE', *, *, #47668, .T. ) ;
#10882=DIRECTION ( 'NONE',  ( -0.7585478161175716050, -0.6516173805718067369, 0.000000000000000000 ) ) ;
#10889=EDGE_CURVE ( 'NONE', #35339, #35674, #8822, .T. ) ;
#10898=CARTESIAN_POINT ( 'NONE',  ( 17.82587367876289974, -104.6869915565625320, -2.500000000000000000 ) ) ;
#10904=EDGE_LOOP ( 'NONE', ( #8343, #33504, #18373, #15885 ) ) ;
#10926=ORIENTED_EDGE ( 'NONE', *, *, #23324, .T. ) ;
#10935=DIRECTION ( 'NONE',  ( -0.9227826878668540234, -0.3853207896976547642, 0.000000000000000000 ) ) ;
#10938=CYLINDRICAL_SURFACE ( 'NONE', #6350, 30.50000000000000000 ) ;
#10942=CARTESIAN_POINT ( 'NONE',  ( 0.6180191030787338669, -93.50720753887522108, -2.500000000000000000 ) ) ;
#10947=EDGE_CURVE ( 'NONE', #12242, #44442, #14943, .T. ) ;
#10950=LINE ( 'NONE', #18536, #27174 ) ;
#10952=DIRECTION ( 'NONE',  ( -0.1045284632676570929, 0.9945218953682730678, 0.000000000000000000 ) ) ;
#10953=DIRECTION ( 'NONE',  ( -0.7273375899149812085, 0.6862798483830533369, 0.000000000000000000 ) ) ;
#10956=PLANE ( 'NONE',  #26875 ) ;
#10957=ADVANCED_FACE ( 'NONE', ( #9543 ), #21538, .F. ) ;
#10967=DIRECTION ( 'NONE',  ( -0.9227826878668540234, -0.3853207896976547642, 0.000000000000000000 ) ) ;
#10969=VERTEX_POINT ( 'NONE', #36463 ) ;
#10970=VERTEX_POINT ( 'NONE', #2927 ) ;
#10975=CARTESIAN_POINT ( 'NONE',  ( -22.67106064244952535, -113.6342314410295842, -2.500000000000000000 ) ) ;
#10997=CARTESIAN_POINT ( 'NONE',  ( -24.50849501662245800, -109.8101191361138831, -5.500000000000000000 ) ) ;
#11007=EDGE_CURVE ( 'NONE', #17038, #29594, #16907, .T. ) ;
#11010=CARTESIAN_POINT ( 'NONE',  ( 19.12409105625795291, -101.5943176906707919, 5.500000000000000000 ) ) ;
#11011=CARTESIAN_POINT ( 'NONE',  ( -21.67772167707813935, -110.8034581014852762, -5.500000000000000000 ) ) ;
#11016=ORIENTED_EDGE ( 'NONE', *, *, #5330, .F. ) ;
#11037=DIRECTION ( 'NONE',  ( -0.6862798483830533369, -0.7273375899149812085, 0.000000000000000000 ) ) ;
#11043=ORIENTED_EDGE ( 'NONE', *, *, #32214, .T. ) ;
#11048=LINE ( 'NONE', #37232, #22661 ) ;
#11067=CARTESIAN_POINT ( 'NONE',  ( -8.826826895187510402, -94.96827758698185562, -2.500000000000000444 ) ) ;
#11070=EDGE_CURVE ( 'NONE', #43520, #17292, #37187, .T. ) ;
#11074=DIRECTION ( 'NONE',  ( -0.000000000000000000, -0.000000000000000000, -1.000000000000000000 ) ) ;
#11082=DIRECTION ( 'NONE',  ( 0.9227826878668540234, 0.3853207896976547087, -0.000000000000000000 ) ) ;
#11093=VECTOR ( 'NONE', #12878, 1000.000000000000114 ) ;
#11110=ORIENTED_EDGE ( 'NONE', *, *, #15088, .T. ) ;
#11120=CARTESIAN_POINT ( 'NONE',  ( -16.06301359042743115, -102.7814171781257357, -2.500000000000000000 ) ) ;
#11126=CARTESIAN_POINT ( 'NONE',  ( -22.53294031248082163, -134.0273518838794757, 2.500000000000000000 ) ) ;
#11131=CARTESIAN_POINT ( 'NONE',  ( 13.83832728059186046, -142.6495187161941089, 5.500000000000000000 ) ) ;
#11138=DIRECTION ( 'NONE',  ( -0.6862798483830534479, -0.7273375899149810975, 0.000000000000000000 ) ) ;
#11144=CARTESIAN_POINT ( 'NONE',  ( 2.117611129180199558, -93.54218975225703048, 5.500000000000000000 ) ) ;
#11147=EDGE_CURVE ( 'NONE', #20756, #42271, #14438, .T. ) ;
#11155=DIRECTION ( 'NONE',  ( 0.9580045777625452175, 0.2867529058022035837, -0.000000000000000000 ) ) ;
#11166=CARTESIAN_POINT ( 'NONE',  ( -23.25244084006223133, -132.7111759872722416, 2.500000000000000000 ) ) ;
#11168=FACE_BOUND ( 'NONE', #1947, .T. ) ;
#11179=CARTESIAN_POINT ( 'NONE',  ( -13.05994868825747446, -139.5943292883446532, 5.500000000000000000 ) ) ;
#11183=( NAMED_UNIT ( * ) PLANE_ANGLE_UNIT ( ) SI_UNIT ( $, .RADIAN. ) );
#11198=DIRECTION ( 'NONE',  ( -0.6862798483830533369, -0.7273375899149812085, 0.000000000000000000 ) ) ;
#11215=ORIENTED_EDGE ( 'NONE', *, *, #23473, .T. ) ;
#11241=AXIS2_PLACEMENT_3D ( 'NONE', #35088, #8182, #8902 ) ;
#11265=VECTOR ( 'NONE', #17675, 1000.000000000000000 ) ;
#11267=DIRECTION ( 'NONE',  ( -0.000000000000000000, -0.000000000000000000, 1.000000000000000000 ) ) ;
#11278=VECTOR ( 'NONE', #9259, 1000.000000000000000 ) ;
#11283=ORIENTED_EDGE ( 'NONE', *, *, #13389, .F. ) ;
#11285=ORIENTED_EDGE ( 'NONE', *, *, #37957, .F. ) ;
#11297=CARTESIAN_POINT ( 'NONE',  ( 9.984461079971730157, -95.40710393340120277, -5.500000000000000000 ) ) ;
#11302=VERTEX_POINT ( 'NONE', #935 ) ;
#11308=DIRECTION ( 'NONE',  ( -0.000000000000000000, -0.000000000000000000, -1.000000000000000000 ) ) ;
#11313=DIRECTION ( 'NONE',  ( -0.7950889364178798102, 0.6064928550163511956, 0.000000000000000000 ) ) ;
#11317=CARTESIAN_POINT ( 'NONE',  ( 19.29194287201271862, -133.5026271600380880, 5.500000000000000000 ) ) ;
#11332=DIRECTION ( 'NONE',  ( 0.9580045777625458836, 0.2867529058022011412, -0.000000000000000000 ) ) ;
#11390=FACE_OUTER_BOUND ( 'NONE', #24022, .T. ) ;
#11397=LINE ( 'NONE', #37078, #23851 ) ;
#11408=VECTOR ( 'NONE', #1361, 1000.000000000000000 ) ;
#11412=EDGE_CURVE ( 'NONE', #35598, #5335, #18216, .T. ) ;
#11415=ADVANCED_FACE ( 'NONE', ( #13177 ), #43038, .F. ) ;
#11421=VERTEX_POINT ( 'NONE', #5846 ) ;
#11422=FACE_OUTER_BOUND ( 'NONE', #27253, .T. ) ;
#11429=ORIENTED_EDGE ( 'NONE', *, *, #9037, .F. ) ;
#11436=LINE ( 'NONE', #45419, #44066 ) ;
#11442=CARTESIAN_POINT ( 'NONE',  ( 16.30584220631899228, -140.9432449716519784, 5.500000000000000000 ) ) ;
#11445=DIRECTION ( 'NONE',  ( 0.9827303690289279636, 0.1850432970638682395, 0.000000000000000000 ) ) ;
#11447=VECTOR ( 'NONE', #22145, 1000.000000000000114 ) ;
#11452=LINE ( 'NONE', #41537, #29141 ) ;
#11453=FACE_OUTER_BOUND ( 'NONE', #16413, .T. ) ;
#11487=EDGE_LOOP ( 'NONE', ( #9784, #35158, #16389, #1221 ) ) ;
#11503=AXIS2_PLACEMENT_3D ( 'NONE', #17196, #24562, #23839 ) ;
#11507=FACE_OUTER_BOUND ( 'NONE', #9570, .T. ) ;
#11511=CARTESIAN_POINT ( 'NONE',  ( -0.7195005275814509993, -118.6838241033926948, 2.500000000000000000 ) ) ;
#11518=CARTESIAN_POINT ( 'NONE',  ( 5.822613034544236399, -142.8165987265839760, 5.500000000000000000 ) ) ;
#11532=ORIENTED_EDGE ( 'NONE', *, *, #43005, .T. ) ;
#11536=CARTESIAN_POINT ( 'NONE',  ( 22.08297821871651934, -111.8242998470044540, -5.500000000000000000 ) ) ;
#11549=DIRECTION ( 'NONE',  ( -0.3311129884571281101, -0.9435911131814402886, 0.000000000000000000 ) ) ;
#11590=VECTOR ( 'NONE', #48123, 1000.000000000000114 ) ;
#11593=EDGE_CURVE ( 'NONE', #15673, #31729, #41475, .T. ) ;
#11600=ORIENTED_EDGE ( 'NONE', *, *, #28083, .T. ) ;
#11607=FACE_OUTER_BOUND ( 'NONE', #781, .T. ) ;
#11610=CARTESIAN_POINT ( 'NONE',  ( -20.30386590532152979, -102.9045904027214959, -5.500000000000000000 ) ) ;
#11613=CARTESIAN_POINT ( 'NONE',  ( -20.30386590532152979, -102.9045904027214959, 5.500000000000000000 ) ) ;
#11621=EDGE_CURVE ( 'NONE', #2795, #40846, #28227, .T. ) ;
#11636=AXIS2_PLACEMENT_3D ( 'NONE', #13959, #6619, #3667 ) ;
#11654=LINE ( 'NONE', #21936, #47274 ) ;
#11657=FACE_OUTER_BOUND ( 'NONE', #36851, .T. ) ;
#11659=CARTESIAN_POINT ( 'NONE',  ( 9.984461079971730157, -95.40710393340120277, 5.500000000000000000 ) ) ;
#11662=DIRECTION ( 'NONE',  ( -0.000000000000000000, -0.000000000000000000, -1.000000000000000000 ) ) ;
#11664=EDGE_CURVE ( 'NONE', #21034, #8377, #45880, .T. ) ;
#11669=LINE ( 'NONE', #41769, #40757 ) ;
#11676=PLANE ( 'NONE',  #7276 ) ;
#11678=DIRECTION ( 'NONE',  ( 0.1850432970638682395, -0.9827303690289279636, 0.000000000000000000 ) ) ;
#11691=CARTESIAN_POINT ( 'NONE',  ( -89.17737905728745318, -39.70432723693717492, 5.500000000000000000 ) ) ;
#11703=DIRECTION ( 'NONE',  ( 0.3311129884571280546, 0.9435911131814402886, 0.000000000000000000 ) ) ;
#11709=ADVANCED_FACE ( 'NONE', ( #5718 ), #4991, .F. ) ;
#11718=EDGE_CURVE ( 'NONE', #39725, #34042, #40458, .T. ) ;
#11720=DIRECTION ( 'NONE',  ( 0.08130631524009970801, -0.9966891607226786576, 0.000000000000000000 ) ) ;
#11726=ORIENTED_EDGE ( 'NONE', *, *, #21495, .T. ) ;
#11732=VERTEX_POINT ( 'NONE', #48025 ) ;
#11740=DIRECTION ( 'NONE',  ( 0.2867529058022035837, -0.9580045777625452175, 0.000000000000000000 ) ) ;
#11749=VERTEX_POINT ( 'NONE', #21835 ) ;
#11803=VECTOR ( 'NONE', #44079, 1000.000000000000000 ) ;
#11806=VERTEX_POINT ( 'NONE', #6205 ) ;
#11817=CARTESIAN_POINT ( 'NONE',  ( 26.09152095774781799, -124.8716048804687375, 5.500000000000000000 ) ) ;
#11827=ORIENTED_EDGE ( 'NONE', *, *, #12906, .F. ) ;
#11886=ORIENTED_EDGE ( 'NONE', *, *, #40599, .T. ) ;
#11894=ORIENTED_EDGE ( 'NONE', *, *, #9995, .T. ) ;
#11913=DIRECTION ( 'NONE',  ( 0.9730327541852497042, -0.2306669878475622604, 0.000000000000000000 ) ) ;
#11920=CARTESIAN_POINT ( 'NONE',  ( -23.30023580412278505, -123.4057321492263384, 5.500000000000000000 ) ) ;
#11932=EDGE_CURVE ( 'NONE', #23907, #14963, #33578, .T. ) ;
#11940=AXIS2_PLACEMENT_3D ( 'NONE', #38520, #37549, #4279 ) ;
#11950=ORIENTED_EDGE ( 'NONE', *, *, #38645, .F. ) ;
#11953=LINE ( 'NONE', #42055, #32548 ) ;
#11986=CARTESIAN_POINT ( 'NONE',  ( -24.94940289813038703, -237.3777120880567963, -5.500000000000000000 ) ) ;
#11995=EDGE_CURVE ( 'NONE', #28510, #46631, #8364, .T. ) ;
#12001=EDGE_CURVE ( 'NONE', #11302, #46719, #38462, .T. ) ;
#12007=ORIENTED_EDGE ( 'NONE', *, *, #43005, .F. ) ;
#12020=VECTOR ( 'NONE', #3499, 1000.000000000000000 ) ;
#12022=FACE_OUTER_BOUND ( 'NONE', #45789, .T. ) ;
#12024=CIRCLE ( 'NONE', #4952, 30.50000000000000000 ) ;
#12026=PLANE ( 'NONE',  #877 ) ;
#12033=CARTESIAN_POINT ( 'NONE',  ( 23.41451323550360186, -132.5004227906269989, -5.500000000000000000 ) ) ;
#12034=ORIENTED_EDGE ( 'NONE', *, *, #6000, .T. ) ;
#12036=CARTESIAN_POINT ( 'NONE',  ( -7.572224309238338336, -145.4393675041377492, 5.500000000000000000 ) ) ;
#12040=DIRECTION ( 'NONE',  ( -0.9038112904824853189, 0.4279312458752976833, 0.000000000000000000 ) ) ;
#12057=VERTEX_POINT ( 'NONE', #46058 ) ;
#12060=VECTOR ( 'NONE', #17090, 1000.000000000000114 ) ;
#12073=EDGE_CURVE ( 'NONE', #35339, #32597, #20100, .T. ) ;
#12082=ORIENTED_EDGE ( 'NONE', *, *, #7528, .T. ) ;
#12100=CARTESIAN_POINT ( 'NONE',  ( 23.49916127795269105, -121.5130826919798039, -2.500000000000000000 ) ) ;
#12103=CARTESIAN_POINT ( 'NONE',  ( 23.30762065077924916, -123.0008031590507329, 2.500000000000000000 ) ) ;
#12109=EDGE_CURVE ( 'NONE', #38735, #47410, #24248, .T. ) ;
#12111=CARTESIAN_POINT ( 'NONE',  ( 23.49916127795269460, -121.5130826919798039, 5.500000000000000000 ) ) ;
#12122=ORIENTED_EDGE ( 'NONE', *, *, #3914, .F. ) ;
#12136=EDGE_CURVE ( 'NONE', #16743, #31838, #4098, .T. ) ;
#12153=ORIENTED_EDGE ( 'NONE', *, *, #9889, .T. ) ;
#12175=DIRECTION ( 'NONE',  ( 0.000000000000000000, 0.000000000000000000, 1.000000000000000000 ) ) ;
#12187=EDGE_CURVE ( 'NONE', #46736, #44017, #23180, .T. ) ;
#12202=CARTESIAN_POINT ( 'NONE',  ( -21.33958957442910886, -129.9559990355020034, 5.500000000000000000 ) ) ;
#12217=DIRECTION ( 'NONE',  ( -0.9227826878668545785, -0.3853207896976533209, 0.000000000000000000 ) ) ;
#12219=PLANE ( 'NONE',  #22759 ) ;
#12242=VERTEX_POINT ( 'NONE', #15369 ) ;
#12255=EDGE_LOOP ( 'NONE', ( #2021, #1152, #9734, #38077 ) ) ;
#12263=ORIENTED_EDGE ( 'NONE', *, *, #41082, .F. ) ;
#12274=LINE ( 'NONE', #12033, #26400 ) ;
#12290=FACE_OUTER_BOUND ( 'NONE', #41017, .T. ) ;
#12299=VERTEX_POINT ( 'NONE', #17029 ) ;
#12304=ORIENTED_EDGE ( 'NONE', *, *, #9761, .T. ) ;
#12308=FACE_OUTER_BOUND ( 'NONE', #23093, .T. ) ;
#12323=CARTESIAN_POINT ( 'NONE',  ( 26.09152095774781799, -124.8716048804687375, 5.500000000000000000 ) ) ;
#12342=DIRECTION ( 'NONE',  ( -0.6064928550163533050, -0.7950889364178781449, 0.000000000000000000 ) ) ;
#12344=DIRECTION ( 'NONE',  ( -0.3311129884571295534, -0.9435911131814398445, 0.000000000000000000 ) ) ;
#12348=EDGE_CURVE ( 'NONE', #29809, #35093, #28061, .T. ) ;
#12352=ORIENTED_EDGE ( 'NONE', *, *, #35778, .F. ) ;
#12388=FACE_OUTER_BOUND ( 'NONE', #48366, .T. ) ;
#12414=PRODUCT_DEFINITION_SHAPE ( 'NONE', 'NONE',  #36966 ) ;
#12418=ORIENTED_EDGE ( 'NONE', *, *, #756, .T. ) ;
#12419=DIRECTION ( 'NONE',  ( 0.6064928550163531940, 0.7950889364178782559, 0.000000000000000000 ) ) ;
#12423=CARTESIAN_POINT ( 'NONE',  ( 26.47460221209471598, -121.8961639463267090, -5.500000000000000000 ) ) ;
#12436=CARTESIAN_POINT ( 'NONE',  ( 21.85433023846371370, -135.0628101570779620, 5.500000000000000000 ) ) ;
#12439=CARTESIAN_POINT ( 'NONE',  ( -10.43921258969510824, -98.89258801967538659, 5.500000000000000000 ) ) ;
#12474=ORIENTED_EDGE ( 'NONE', *, *, #38695, .F. ) ;
#12495=DIRECTION ( 'NONE',  ( 0.000000000000000000, 0.000000000000000000, 1.000000000000000000 ) ) ;
#12496=AXIS2_PLACEMENT_3D ( 'NONE', #39814, #25586, #43488 ) ;
#12500=COLOUR_RGB ( '', 0.08235294, 0.09019608, 0.10196078) ;
#12509=ORIENTED_EDGE ( 'NONE', *, *, #23657, .T. ) ;
#12523=CARTESIAN_POINT ( 'NONE',  ( -26.53422223201112828, -120.6595836127786043, 5.500000000000000000 ) ) ;
#12532=CARTESIAN_POINT ( 'NONE',  ( -12.50000000000000000, -107.5000000000000000, 2.500000000000000000 ) ) ;
#12536=VECTOR ( 'NONE', #36716, 1000.000000000000000 ) ;
#12542=VECTOR ( 'NONE', #44280, 1000.000000000000000 ) ;
#12543=FACE_OUTER_BOUND ( 'NONE', #16882, .T. ) ;
#12549=VERTEX_POINT ( 'NONE', #29003 ) ;
#12552=EDGE_LOOP ( 'NONE', ( #28037, #46867, #32553, #14547 ) ) ;
#12553=CARTESIAN_POINT ( 'NONE',  ( 24.95699195200416654, -110.9640411295978595, 5.500000000000000000 ) ) ;
#12554=EDGE_CURVE ( 'NONE', #21021, #3684, #37076, .T. ) ;
#12561=ORIENTED_EDGE ( 'NONE', *, *, #39079, .F. ) ;
#12582=DIRECTION ( 'NONE',  ( -0.000000000000000000, -0.000000000000000000, -1.000000000000000000 ) ) ;
#12588=ORIENTED_EDGE ( 'NONE', *, *, #1610, .T. ) ;
#12589=VERTEX_POINT ( 'NONE', #4756 ) ;
#12617=ORIENTED_EDGE ( 'NONE', *, *, #7410, .T. ) ;
#12622=CARTESIAN_POINT ( 'NONE',  ( 2.047646702416564768, -96.54137380445985173, -5.500000000000000000 ) ) ;
#12633=ADVANCED_FACE ( 'NONE', ( #30963 ), #45627, .F. ) ;
#12634=CARTESIAN_POINT ( 'NONE',  ( -25.50183398199384754, -112.6408924756582053, 5.500000000000000000 ) ) ;
#12648=CARTESIAN_POINT ( 'NONE',  ( -0.8815729230226008184, -93.47222532549339746, 5.500000000000000000 ) ) ;
#12702=CIRCLE ( 'NONE', #39251, 35.50000000000000711 ) ;
#12704=LINE ( 'NONE', #16376, #37948 ) ;
#12729=VERTEX_POINT ( 'NONE', #2065 ) ;
#12746=EDGE_LOOP ( 'NONE', ( #25637, #33473, #22950, #20560 ) ) ;
#12757=EDGE_CURVE ( 'NONE', #12729, #15261, #46843, .T. ) ;
#12776=AXIS2_PLACEMENT_3D ( 'NONE', #13645, #25609, #32490 ) ;
#12777=FACE_OUTER_BOUND ( 'NONE', #25289, .T. ) ;
#12791=DIRECTION ( 'NONE',  ( -0.000000000000000000, -0.000000000000000000, -1.000000000000000000 ) ) ;
#12796=DIRECTION ( 'NONE',  ( 0.9580045777625458836, 0.2867529058022011412, 0.000000000000000000 ) ) ;
#12812=DIRECTION ( 'NONE',  ( 0.4796670183876317051, -0.8774505977381971134, 0.000000000000000000 ) ) ;
#12825=AXIS2_PLACEMENT_3D ( 'NONE', #25732, #40673, #273 ) ;
#12828=DIRECTION ( 'NONE',  ( 0.7950889364178796992, -0.6064928550163510845, 0.000000000000000000 ) ) ;
#12839=EDGE_CURVE ( 'NONE', #43487, #21261, #20646, .T. ) ;
#12856=DIRECTION ( 'NONE',  ( 0.2306669878475637314, 0.9730327541852493711, 0.000000000000000000 ) ) ;
#12859=ORIENTED_EDGE ( 'NONE', *, *, #23657, .F. ) ;
#12866=CARTESIAN_POINT ( 'NONE',  ( -17.26469406256017791, -140.1601175325492648, 5.500000000000000000 ) ) ;
#12867=ORIENTED_EDGE ( 'NONE', *, *, #20898, .F. ) ;
#12878=DIRECTION ( 'NONE',  ( -0.9730327541852497042, 0.2306669878475623159, 0.000000000000000000 ) ) ;
#12905=EDGE_LOOP ( 'NONE', ( #5275, #12122, #1140, #32700 ) ) ;
#12906=EDGE_CURVE ( 'NONE', #28234, #46631, #25754, .T. ) ;
#12913=VECTOR ( 'NONE', #27384, 1000.000000000000000 ) ;
#12929=EDGE_LOOP ( 'NONE', ( #27132, #39761, #8839, #32115 ) ) ;
#12931=DIRECTION ( 'NONE',  ( -0.000000000000000000, -0.000000000000000000, -1.000000000000000000 ) ) ;
#12954=ADVANCED_FACE ( 'NONE', ( #48037 ), #29194, .T. ) ;
#12967=ORIENTED_EDGE ( 'NONE', *, *, #42773, .T. ) ;
#12968=ORIENTED_EDGE ( 'NONE', *, *, #11664, .F. ) ;
#12987=DIRECTION ( 'NONE',  ( 0.1850432970638656582, -0.9827303690289285187, 0.000000000000000000 ) ) ;
#13009=CARTESIAN_POINT ( 'NONE',  ( -103.9230484541323705, -180.0000000000004832, -5.500000000000000000 ) ) ;
#13019=LINE ( 'NONE', #20102, #20537 ) ;
#13022=FACE_OUTER_BOUND ( 'NONE', #6425, .T. ) ;
#13029=CARTESIAN_POINT ( 'NONE',  ( 0.4966694826857007139, -118.5846133302278247, 2.500000000000000000 ) ) ;
#13044=ORIENTED_EDGE ( 'NONE', *, *, #3501, .F. ) ;
#13051=DIRECTION ( 'NONE',  ( 0.000000000000000000, 0.000000000000000000, 1.000000000000000000 ) ) ;
#13092=ADVANCED_FACE ( 'NONE', ( #15001 ), #42144, .F. ) ;
#13103=VECTOR ( 'NONE', #283, 999.9999999999998863 ) ;
#13105=DIRECTION ( 'NONE',  ( 0.2306669878475623159, 0.9730327541852497042, -0.000000000000000000 ) ) ;
#13109=DIRECTION ( 'NONE',  ( -0.8774505977381983346, -0.4796670183876294291, 0.000000000000000000 ) ) ;
#13125=DIRECTION ( 'NONE',  ( 0.5200609990132993854, 0.8541291221503275466, -0.000000000000000000 ) ) ;
#13169=EDGE_CURVE ( 'NONE', #12299, #9209, #2010, .T. ) ;
#13170=LINE ( 'NONE', #42797, #3984 ) ;
#13175=ORIENTED_EDGE ( 'NONE', *, *, #26594, .T. ) ;
#13176=CARTESIAN_POINT ( 'NONE',  ( 2.047646702416564768, -96.54137380445985173, 2.500000000000000000 ) ) ;
#13177=FACE_OUTER_BOUND ( 'NONE', #39704, .T. ) ;
#13203=FACE_OUTER_BOUND ( 'NONE', #12746, .T. ) ;
#13208=VERTEX_POINT ( 'NONE', #43112 ) ;
#13213=CARTESIAN_POINT ( 'NONE',  ( 2.874421927457452952, -143.3717286177755739, -2.500000000000000000 ) ) ;
#13218=ORIENTED_EDGE ( 'NONE', *, *, #30848, .T. ) ;
#13231=VERTEX_POINT ( 'NONE', #1753 ) ;
#13235=CARTESIAN_POINT ( 'NONE',  ( -15.44521549751111422, -137.7748507232956001, 5.500000000000000000 ) ) ;
#13236=DIRECTION ( 'NONE',  ( -0.000000000000000000, -0.000000000000000000, -1.000000000000000000 ) ) ;
#13239=DIRECTION ( 'NONE',  ( 0.000000000000000000, 0.000000000000000000, 1.000000000000000000 ) ) ;
#13246=CARTESIAN_POINT ( 'NONE',  ( -26.53422223201112828, -120.6595836127786043, 2.500000000000000000 ) ) ;
#13258=EDGE_LOOP ( 'NONE', ( #27782, #22358, #22819, #8781 ) ) ;
#13263=VERTEX_POINT ( 'NONE', #15372 ) ;
#13274=DIRECTION ( 'NONE',  ( -0.000000000000000000, -0.000000000000000000, -1.000000000000000000 ) ) ;
#13275=ORIENTED_EDGE ( 'NONE', *, *, #47665, .F. ) ;
#13278=FACE_BOUND ( 'NONE', #20861, .T. ) ;
#13279=CARTESIAN_POINT ( 'NONE',  ( 21.85433023846371370, -135.0628101570779620, 5.500000000000000000 ) ) ;
#13322=EDGE_CURVE ( 'NONE', #42528, #14101, #171, .T. ) ;
#13323=VECTOR ( 'NONE', #18728, 1000.000000000000000 ) ;
#13336=CARTESIAN_POINT ( 'NONE',  ( -7.572224309238338336, -145.4393675041377492, 5.500000000000000000 ) ) ;
#13347=LINE ( 'NONE', #2551, #21463 ) ;
#13368=VECTOR ( 'NONE', #34333, 1000.000000000000000 ) ;
#13389=EDGE_CURVE ( 'NONE', #28753, #22152, #15836, .T. ) ;
#13401=VECTOR ( 'NONE', #448, 1000.000000000000000 ) ;
#13423=LINE ( 'NONE', #43531, #45614 ) ;
#13431=ORIENTED_EDGE ( 'NONE', *, *, #7578, .T. ) ;
#13434=VECTOR ( 'NONE', #8868, 1000.000000000000114 ) ;
#13444=DIRECTION ( 'NONE',  ( -0.8225049752423791993, -0.5687579148473745905, 0.000000000000000000 ) ) ;
#13446=ORIENTED_EDGE ( 'NONE', *, *, #47671, .T. ) ;
#13455=DIRECTION ( 'NONE',  ( -0.9966891607226786576, -0.08130631524009861166, 0.000000000000000000 ) ) ;
#13458=ORIENTED_EDGE ( 'NONE', *, *, #30304, .T. ) ;
#13472=VECTOR ( 'NONE', #10882, 1000.000000000000000 ) ;
#13481=DIRECTION ( 'NONE',  ( 0.1850432970638656860, -0.9827303690289285187, 0.000000000000000000 ) ) ;
#13484=EDGE_LOOP ( 'NONE', ( #43557, #44261, #35568, #27656 ) ) ;
#13535=LINE ( 'NONE', #17916, #8249 ) ;
#13541=PLANE ( 'NONE',  #18158 ) ;
#13549=ORIENTED_EDGE ( 'NONE', *, *, #14026, .T. ) ;
#13553=DIRECTION ( 'NONE',  ( -0.000000000000000000, -0.000000000000000000, -1.000000000000000000 ) ) ;
#13557=ORIENTED_EDGE ( 'NONE', *, *, #45166, .T. ) ;
#13585=DIRECTION ( 'NONE',  ( -0.4279312458752990711, -0.9038112904824846527, 0.000000000000000000 ) ) ;
#13597=EDGE_CURVE ( 'NONE', #10091, #14358, #43482, .T. ) ;
#13607=VECTOR ( 'NONE', #45669, 1000.000000000000000 ) ;
#13610=ORIENTED_EDGE ( 'NONE', *, *, #12187, .T. ) ;
#13612=EDGE_LOOP ( 'NONE', ( #37721, #15785, #13770, #47575 ) ) ;
#13616=VECTOR ( 'NONE', #18086, 1000.000000000000000 ) ;
#13633=VECTOR ( 'NONE', #1496, 999.9999999999998863 ) ;
#13638=PLANE ( 'NONE',  #26301 ) ;
#13645=CARTESIAN_POINT ( 'NONE',  ( 0.000000000000000000, -120.0000000000000000, -2.500000000000000000 ) ) ;
#13677=EDGE_CURVE ( 'NONE', #15673, #24295, #17982, .T. ) ;
#13688=LINE ( 'NONE', #40829, #6971 ) ;
#13694=LINE ( 'NONE', #14169, #1632 ) ;
#13744=DIRECTION ( 'NONE',  ( -0.000000000000000000, -0.000000000000000000, -1.000000000000000000 ) ) ;
#13757=LINE ( 'NONE', #35781, #15659 ) ;
#13770=ORIENTED_EDGE ( 'NONE', *, *, #17179, .T. ) ;
#13792=EDGE_CURVE ( 'NONE', #13231, #28317, #10413, .T. ) ;
#13796=CARTESIAN_POINT ( 'NONE',  ( 1.192633404626820770, -120.9097392825245407, -2.500000000000000000 ) ) ;
#13804=VECTOR ( 'NONE', #537, 1000.000000000000114 ) ;
#13813=AXIS2_PLACEMENT_3D ( 'NONE', #21725, #28824, #32730 ) ;
#13815=AXIS2_PLACEMENT_3D ( 'NONE', #32976, #44248, #10952 ) ;
#13820=CARTESIAN_POINT ( 'NONE',  ( 8.700667342345820288, -98.11853780484867116, -2.500000000000000000 ) ) ;
#13824=ORIENTED_EDGE ( 'NONE', *, *, #30546, .T. ) ;
#13842=CARTESIAN_POINT ( 'NONE',  ( -12.50000000000000000, -107.5000000000000000, -2.500000000000000000 ) ) ;
#13846=DIRECTION ( 'NONE',  ( 0.08130631524010120681, -0.9966891607226784355, 0.000000000000000000 ) ) ;
#13871=ORIENTED_EDGE ( 'NONE', *, *, #41936, .T. ) ;
#13875=CARTESIAN_POINT ( 'NONE',  ( -0.4966694826856976608, -121.4153866697721611, 2.500000000000000000 ) ) ;
#13901=FACE_OUTER_BOUND ( 'NONE', #6392, .T. ) ;
#13903=LINE ( 'NONE', #17806, #23256 ) ;
#13905=PLANE ( 'NONE',  #6792 ) ;
#13906=CARTESIAN_POINT ( 'NONE',  ( -13.05994868825747446, -139.5943292883446532, 5.500000000000000000 ) ) ;
#13920=ORIENTED_EDGE ( 'NONE', *, *, #32356, .T. ) ;
#13934=PRODUCT_DEFINITION_FORMATION_WITH_SPECIFIED_SOURCE ( 'ANY', '', #40211, .NOT_KNOWN. ) ;
#13936=VERTEX_POINT ( 'NONE', #38541 ) ;
#13938=ORIENTED_EDGE ( 'NONE', *, *, #39699, .F. ) ;
#13946=ORIENTED_EDGE ( 'NONE', *, *, #5209, .T. ) ;
#13959=CARTESIAN_POINT ( 'NONE',  ( 0.000000000000000000, 0.000000000000000000, 0.000000000000000000 ) ) ;
#13979=VERTEX_POINT ( 'NONE', #39514 ) ;
#13991=VECTOR ( 'NONE', #22369, 1000.000000000000000 ) ;
#13994=CARTESIAN_POINT ( 'NONE',  ( 103.9230484541331947, -179.9999999999990337, -5.500000000000000000 ) ) ;
#14008=DIRECTION ( 'NONE',  ( -0.6862798483830533369, -0.7273375899149812085, 0.000000000000000000 ) ) ;
#14014=CARTESIAN_POINT ( 'NONE',  ( -0.9515373497862389396, -96.47140937769621871, -2.500000000000000000 ) ) ;
#14024=ORIENTED_EDGE ( 'NONE', *, *, #15541, .F. ) ;
#14026=EDGE_CURVE ( 'NONE', #5563, #28753, #42937, .T. ) ;
#14030=CARTESIAN_POINT ( 'NONE',  ( 12.69589495141918611, -96.69089767102708777, -5.500000000000000000 ) ) ;
#14049=ORIENTED_EDGE ( 'NONE', *, *, #9174, .T. ) ;
#14051=DIRECTION ( 'NONE',  ( 0.000000000000000000, 0.000000000000000000, -1.000000000000000000 ) ) ;
#14062=DIRECTION ( 'NONE',  ( -0.000000000000000000, -0.000000000000000000, 1.000000000000000000 ) ) ;
#14076=DIRECTION ( 'NONE',  ( -0.000000000000000000, -0.000000000000000000, 1.000000000000000000 ) ) ;
#14083=FACE_OUTER_BOUND ( 'NONE', #39569, .T. ) ;
#14101=VERTEX_POINT ( 'NONE', #47788 ) ;
#14102=CARTESIAN_POINT ( 'NONE',  ( -5.420674214417706693, -142.8662697233533265, -2.500000000000000000 ) ) ;
#14108=CARTESIAN_POINT ( 'NONE',  ( -4.653126046682595884, -146.1313684676804314, 5.500000000000000000 ) ) ;
#14112=CARTESIAN_POINT ( 'NONE',  ( 2.874421927457452952, -143.3717286177755739, -5.500000000000000000 ) ) ;
#14146=CARTESIAN_POINT ( 'NONE',  ( -22.53294031248082163, -134.0273518838794757, 5.500000000000000000 ) ) ;
#14150=LINE ( 'NONE', #37385, #2642 ) ;
#14158=LINE ( 'NONE', #14650, #15969 ) ;
#14159=ORIENTED_EDGE ( 'NONE', *, *, #34146, .T. ) ;
#14167=ORIENTED_EDGE ( 'NONE', *, *, #7125, .T. ) ;
#14169=CARTESIAN_POINT ( 'NONE',  ( 22.94323693612312809, -114.6983135802921083, 5.500000000000000000 ) ) ;
#14178=ORIENTED_EDGE ( 'NONE', *, *, #21619, .T. ) ;
#14197=DIRECTION ( 'NONE',  ( -0.000000000000000000, -0.000000000000000000, -1.000000000000000000 ) ) ;
#14208=EDGE_CURVE ( 'NONE', #14101, #7679, #36776, .T. ) ;
#14221=DIRECTION ( 'NONE',  ( -0.9580045777625452175, -0.2867529058022035837, 0.000000000000000000 ) ) ;
#14223=LINE ( 'NONE', #17883, #2378 ) ;
#14229=ORIENTED_EDGE ( 'NONE', *, *, #555, .T. ) ;
#14234=CARTESIAN_POINT ( 'NONE',  ( -21.33958957442910886, -129.9559990355020034, -5.500000000000000000 ) ) ;
#14239=VERTEX_POINT ( 'NONE', #1021 ) ;
#14242=ORIENTED_EDGE ( 'NONE', *, *, #21251, .F. ) ;
#14250=CARTESIAN_POINT ( 'NONE',  ( -26.29030328629083968, -123.6496510949466341, 5.500000000000000000 ) ) ;
#14255=CARTESIAN_POINT ( 'NONE',  ( -114.1267819554185365, -82.91796067500661138, -5.500000000000000000 ) ) ;
#14270=ORIENTED_EDGE ( 'NONE', *, *, #42992, .F. ) ;
#14275=CARTESIAN_POINT ( 'NONE',  ( 11.41210121379328335, -99.40233154247455616, 5.500000000000000000 ) ) ;
#14296=ADVANCED_FACE ( 'NONE', ( #12308 ), #34074, .F. ) ;
#14300=ORIENTED_EDGE ( 'NONE', *, *, #46052, .T. ) ;
#14303=DIRECTION ( 'NONE',  ( -0.000000000000000000, -0.000000000000000000, -1.000000000000000000 ) ) ;
#14313=FACE_OUTER_BOUND ( 'NONE', #1747, .T. ) ;
#14315=EDGE_LOOP ( 'NONE', ( #20847, #8853, #46143, #7479 ) ) ;
#14327=AXIS2_PLACEMENT_3D ( 'NONE', #16927, #21063, #32104 ) ;
#14354=VECTOR ( 'NONE', #30360, 1000.000000000000000 ) ;
#14358=VERTEX_POINT ( 'NONE', #26739 ) ;
#14359=ORIENTED_EDGE ( 'NONE', *, *, #34114, .F. ) ;
#14361=EDGE_LOOP ( 'NONE', ( #47044, #6334, #33842, #6309 ) ) ;
#14365=FACE_BOUND ( 'NONE', #11487, .T. ) ;
#14374=LINE ( 'NONE', #40799, #34525 ) ;
#14377=ADVANCED_FACE ( 'NONE', ( #12777 ), #42882, .F. ) ;
#14379=AXIS2_PLACEMENT_3D ( 'NONE', #29481, #18207, #33396 ) ;
#14424=AXIS2_PLACEMENT_3D ( 'NONE', #42016, #31739, #27086 ) ;
#14438=LINE ( 'NONE', #8525, #2105 ) ;
#14451=DIRECTION ( 'NONE',  ( -0.000000000000000000, -0.000000000000000000, -1.000000000000000000 ) ) ;
#14453=ORIENTED_EDGE ( 'NONE', *, *, #18827, .F. ) ;
#14461=CARTESIAN_POINT ( 'NONE',  ( -25.50183398199384754, -112.6408924756582053, -5.500000000000000000 ) ) ;
#14467=LINE ( 'NONE', #40890, #33108 ) ;
#14468=ORIENTED_EDGE ( 'NONE', *, *, #26594, .F. ) ;
#14473=CARTESIAN_POINT ( 'NONE',  ( -16.06301359042743115, -102.7814171781257357, 5.500000000000000000 ) ) ;
#14474=ORIENTED_EDGE ( 'NONE', *, *, #2960, .T. ) ;
#14480=EDGE_CURVE ( 'NONE', #3370, #16986, #6157, .T. ) ;
#14492=ORIENTED_EDGE ( 'NONE', *, *, #12348, .T. ) ;
#14503=ORIENTED_EDGE ( 'NONE', *, *, #9176, .T. ) ;
#14510=DIRECTION ( 'NONE',  ( -0.08130631524010117905, 0.9966891607226784355, 0.000000000000000000 ) ) ;
#14518=ORIENTED_EDGE ( 'NONE', *, *, #4151, .T. ) ;
#14536=VECTOR ( 'NONE', #15999, 1000.000000000000000 ) ;
#14540=DIRECTION ( 'NONE',  ( 0.5687579148473752566, -0.8225049752423786442, 0.000000000000000000 ) ) ;
#14544=EDGE_LOOP ( 'NONE', ( #1965, #34852, #35760, #38429 ) ) ;
#14547=ORIENTED_EDGE ( 'NONE', *, *, #32647, .T. ) ;
#14550=EDGE_CURVE ( 'NONE', #38166, #44442, #18108, .T. ) ;
#14558=ORIENTED_EDGE ( 'NONE', *, *, #29185, .F. ) ;
#14574=EDGE_CURVE ( 'NONE', #44487, #30240, #47973, .T. ) ;
#14578=DIRECTION ( 'NONE',  ( -0.7585478161175723821, -0.6516173805718057377, 0.000000000000000000 ) ) ;
#14583=DIRECTION ( 'NONE',  ( -0.8774505977381978905, -0.4796670183876304283, 0.000000000000000000 ) ) ;
#14593=VERTEX_POINT ( 'NONE', #14461 ) ;
#14606=ORIENTED_EDGE ( 'NONE', *, *, #8602, .T. ) ;
#14610=LINE ( 'NONE', #6529, #2984 ) ;
#14616=DIRECTION ( 'NONE',  ( -0.4796670183876317051, 0.8774505977381971134, 0.000000000000000000 ) ) ;
#14623=DIRECTION ( 'NONE',  ( -0.2306669878475637314, -0.9730327541852493711, 0.000000000000000000 ) ) ;
#14633=ORIENTED_EDGE ( 'NONE', *, *, #29606, .T. ) ;
#14638=AXIS2_PLACEMENT_3D ( 'NONE', #28752, #13105, #2092 ) ;
#14640=PLANE ( 'NONE',  #2655 ) ;
#14650=CARTESIAN_POINT ( 'NONE',  ( 22.51310757741980240, -113.2613067136482101, 2.500000000000000000 ) ) ;
#14660=PLANE ( 'NONE',  #30549 ) ;
#14669=ORIENTED_EDGE ( 'NONE', *, *, #39973, .F. ) ;
#14679=EDGE_LOOP ( 'NONE', ( #4087, #19986, #2300, #16732 ) ) ;
#14681=LINE ( 'NONE', #43804, #22998 ) ;
#14687=PLANE ( 'NONE',  #42731 ) ;
#14689=PLANE ( 'NONE',  #47323 ) ;
#14700=EDGE_CURVE ( 'NONE', #18493, #25478, #4418, .T. ) ;
#14711=ORIENTED_EDGE ( 'NONE', *, *, #2251, .F. ) ;
#14713=ORIENTED_EDGE ( 'NONE', *, *, #18169, .F. ) ;
#14724=ORIENTED_EDGE ( 'NONE', *, *, #19897, .T. ) ;
#14736=CARTESIAN_POINT ( 'NONE',  ( -17.26469406256017791, -140.1601175325492648, 5.500000000000000000 ) ) ;
#14738=CARTESIAN_POINT ( 'NONE',  ( 20.85212586905262100, -130.9402397935870965, 5.500000000000000000 ) ) ;
#14743=CARTESIAN_POINT ( 'NONE',  ( 12.69589495141918611, -96.69089767102708777, 5.500000000000000000 ) ) ;
#14760=DIRECTION ( 'NONE',  ( -0.4999999999999919509, -0.8660254037844432595, 0.000000000000000000 ) ) ;
#14777=ORIENTED_EDGE ( 'NONE', *, *, #29724, .F. ) ;
#14799=CARTESIAN_POINT ( 'NONE',  ( 0.9774260708577211521, -121.1378217241763622, 2.500000000000000000 ) ) ;
#14800=LINE ( 'NONE', #44898, #42662 ) ;
#14814=CARTESIAN_POINT ( 'NONE',  ( 3.429551818649054340, -146.3199197248623875, 5.500000000000000000 ) ) ;
#14818=ADVANCED_FACE ( 'NONE', ( #45278 ), #39143, .F. ) ;
#14821=EDGE_CURVE ( 'NONE', #29948, #28234, #19795, .T. ) ;
#14833=DIRECTION ( 'NONE',  ( -0.6516173805718079581, 0.7585478161175704948, 0.000000000000000000 ) ) ;
#14837=LINE ( 'NONE', #40536, #13323 ) ;
#14840=ORIENTED_EDGE ( 'NONE', *, *, #6568, .F. ) ;
#14848=VERTEX_POINT ( 'NONE', #27408 ) ;
#14850=DIRECTION ( 'NONE',  ( 0.7273375899149812085, -0.6862798483830533369, 0.000000000000000000 ) ) ;
#14855=DIRECTION ( 'NONE',  ( 1.000000000000000000, 0.000000000000000000, 0.000000000000000000 ) ) ;
#14879=ADVANCED_FACE ( 'NONE', ( #31328 ), #32051, .F. ) ;
#14892=VECTOR ( 'NONE', #29029, 1000.000000000000114 ) ;
#14896=ORIENTED_EDGE ( 'NONE', *, *, #25767, .F. ) ;
#14918=LINE ( 'NONE', #29366, #29233 ) ;
#14924=CARTESIAN_POINT ( 'NONE',  ( 1.499592026101426168, -120.0349822133818094, -2.500000000000000000 ) ) ;
#14943=CIRCLE ( 'NONE', #40720, 30.50000000000000000 ) ;
#14947=VERTEX_POINT ( 'NONE', #21013 ) ;
#14963=VERTEX_POINT ( 'NONE', #32745 ) ;
#14965=LINE ( 'NONE', #40437, #31275 ) ;
#14979=CARTESIAN_POINT ( 'NONE',  ( 2.874421927457452952, -143.3717286177755739, 5.500000000000000000 ) ) ;
#14991=EDGE_CURVE ( 'NONE', #36404, #11421, #14158, .T. ) ;
#15001=FACE_OUTER_BOUND ( 'NONE', #29578, .T. ) ;
#15017=DIRECTION ( 'NONE',  ( 0.000000000000000000, -0.000000000000000000, 1.000000000000000000 ) ) ;
#15041=AXIS2_PLACEMENT_3D ( 'NONE', #28055, #31493, #27567 ) ;
#15043=LINE ( 'NONE', #11613, #34816 ) ;
#15053=CARTESIAN_POINT ( 'NONE',  ( -0.9515373497862389396, -96.47140937769621871, 5.500000000000000000 ) ) ;
#15074=VECTOR ( 'NONE', #4128, 1000.000000000000114 ) ;
#15082=ORIENTED_EDGE ( 'NONE', *, *, #39800, .F. ) ;
#15088=EDGE_CURVE ( 'NONE', #32597, #17971, #40109, .T. ) ;
#15111=CARTESIAN_POINT ( 'NONE',  ( 25.81725066941077529, -113.8380548628854854, -2.500000000000000444 ) ) ;
#15131=ORIENTED_EDGE ( 'NONE', *, *, #46007, .T. ) ;
#15140=PLANE ( 'NONE',  #2249 ) ;
#15155=EDGE_CURVE ( 'NONE', #23903, #7237, #41086, .T. ) ;
#15156=ORIENTED_EDGE ( 'NONE', *, *, #33378, .T. ) ;
#15157=CARTESIAN_POINT ( 'NONE',  ( 13.83832728059186046, -142.6495187161941089, -5.500000000000000000 ) ) ;
#15170=DIRECTION ( 'NONE',  ( -0.5200609990132993854, -0.8541291221503275466, 0.000000000000000000 ) ) ;
#15180=PLANE ( 'NONE',  #39711 ) ;
#15190=EDGE_LOOP ( 'NONE', ( #35102, #31503, #29389, #28518 ) ) ;
#15214=LINE ( 'NONE', #29413, #35439 ) ;
#15226=VECTOR ( 'NONE', #39782, 1000.000000000000000 ) ;
#15240=DIRECTION ( 'NONE',  ( -1.000000000000000000, 0.000000000000000000, -0.000000000000000000 ) ) ;
#15259=CARTESIAN_POINT ( 'NONE',  ( 9.984461079971730157, -95.40710393340120277, 5.500000000000000000 ) ) ;
#15261=VERTEX_POINT ( 'NONE', #28731 ) ;
#15266=EDGE_CURVE ( 'NONE', #17111, #15663, #6455, .T. ) ;
#15272=VECTOR ( 'NONE', #43457, 1000.000000000000000 ) ;
#15293=DIRECTION ( 'NONE',  ( 1.000000000000000000, 0.000000000000000000, 0.000000000000000000 ) ) ;
#15296=DIRECTION ( 'NONE',  ( -0.7950889364178798102, 0.6064928550163511956, 0.000000000000000000 ) ) ;
#15312=ORIENTED_EDGE ( 'NONE', *, *, #8337, .T. ) ;
#15320=ORIENTED_EDGE ( 'NONE', *, *, #47188, .F. ) ;
#15327=FACE_OUTER_BOUND ( 'NONE', #23350, .T. ) ;
#15334=PLANE ( 'NONE',  #19373 ) ;
#15336=DIRECTION ( 'NONE',  ( -0.5200609990132993854, -0.8541291221503275466, 0.000000000000000000 ) ) ;
#15347=DIRECTION ( 'NONE',  ( 0.000000000000000000, 0.000000000000000000, 1.000000000000000000 ) ) ;
#15352=LINE ( 'NONE', #25850, #25344 ) ;
#15353=EDGE_LOOP ( 'NONE', ( #34220, #41108 ) ) ;
#15366=CARTESIAN_POINT ( 'NONE',  ( 19.12409105625795291, -101.5943176906707919, 5.500000000000000000 ) ) ;
#15369=CARTESIAN_POINT ( 'NONE',  ( 30.50000000000000000, -120.0000000000000000, -2.500000000000000000 ) ) ;
#15372=CARTESIAN_POINT ( 'NONE',  ( -26.29030328629083968, -123.6496510949466341, 2.500000000000000000 ) ) ;
#15380=DIRECTION ( 'NONE',  ( 0.9966891607226786576, 0.08130631524009862554, 0.000000000000000000 ) ) ;
#15411=DIRECTION ( 'NONE',  ( -0.8774505977381983346, -0.4796670183876294291, 0.000000000000000000 ) ) ;
#15421=FACE_OUTER_BOUND ( 'NONE', #21760, .T. ) ;
#15449=ORIENTED_EDGE ( 'NONE', *, *, #39034, .T. ) ;
#15458=EDGE_LOOP ( 'NONE', ( #26724, #30001, #19374, #38143 ) ) ;
#15459=CARTESIAN_POINT ( 'NONE',  ( -11.59517495878806947, -96.12423995607481686, 5.500000000000000000 ) ) ;
#15460=LINE ( 'NONE', #34517, #38687 ) ;
#15494=VECTOR ( 'NONE', #9302, 1000.000000000000000 ) ;
#15504=LINE ( 'NONE', #45346, #13991 ) ;
#15516=DIRECTION ( 'NONE',  ( 0.1276937514489679404, 0.9918136447140103451, -0.000000000000000000 ) ) ;
#15524=CARTESIAN_POINT ( 'NONE',  ( -18.24502636017238899, -100.7225776329765665, 5.500000000000000000 ) ) ;
#15526=ADVANCED_FACE ( 'NONE', ( #12543 ), #38483, .F. ) ;
#15539=EDGE_CURVE ( 'NONE', #44487, #47761, #34548, .T. ) ;
#15541=EDGE_CURVE ( 'NONE', #30085, #41259, #37759, .T. ) ;
#15565=LINE ( 'NONE', #12622, #40506 ) ;
#15581=LINE ( 'NONE', #45934, #10543 ) ;
#15586=DIRECTION ( 'NONE',  ( 0.000000000000000000, 0.000000000000000000, 1.000000000000000000 ) ) ;
#15623=ORIENTED_EDGE ( 'NONE', *, *, #33977, .T. ) ;
#15628=ORIENTED_EDGE ( 'NONE', *, *, #32656, .F. ) ;
#15629=VECTOR ( 'NONE', #22592, 1000.000000000000000 ) ;
#15635=CARTESIAN_POINT ( 'NONE',  ( -23.54415474984308787, -120.4156646670583086, 2.500000000000000000 ) ) ;
#15644=LINE ( 'NONE', #41360, #9100 ) ;
#15652=ORIENTED_EDGE ( 'NONE', *, *, #7890, .T. ) ;
#15659=VECTOR ( 'NONE', #47284, 1000.000000000000114 ) ;
#15663=VERTEX_POINT ( 'NONE', #38978 ) ;
#15673=VERTEX_POINT ( 'NONE', #35046 ) ;
#15679=CARTESIAN_POINT ( 'NONE',  ( 2.117611129180199558, -93.54218975225703048, 5.500000000000000000 ) ) ;
#15690=DIRECTION ( 'NONE',  ( 0.7273375899149802093, -0.6862798483830544471, 0.000000000000000000 ) ) ;
#15692=CARTESIAN_POINT ( 'NONE',  ( -30.50000000000000000, -120.0000000000000000, 2.500000000000000000 ) ) ;
#15705=EDGE_LOOP ( 'NONE', ( #25401, #47493, #14474, #36014 ) ) ;
#15713=EDGE_LOOP ( 'NONE', ( #47476, #41385, #26259, #45866 ) ) ;
#15731=DIRECTION ( 'NONE',  ( -0.000000000000000000, -0.000000000000000000, -1.000000000000000000 ) ) ;
#15747=ORIENTED_EDGE ( 'NONE', *, *, #2808, .F. ) ;
#15755=CARTESIAN_POINT ( 'NONE',  ( 25.81725066941077529, -113.8380548628854854, 5.500000000000000000 ) ) ;
#15760=CARTESIAN_POINT ( 'NONE',  ( 1.192633404626820770, -120.9097392825245407, 2.500000000000000000 ) ) ;
#15779=VECTOR ( 'NONE', #15336, 1000.000000000000114 ) ;
#15785=ORIENTED_EDGE ( 'NONE', *, *, #17071, .T. ) ;
#15798=EDGE_CURVE ( 'NONE', #12057, #3234, #14467, .T. ) ;
#15813=CARTESIAN_POINT ( 'NONE',  ( 0.7800914985199594032, -118.7188063167744900, 2.500000000000000000 ) ) ;
#15821=LINE ( 'NONE', #12634, #412 ) ;
#15825=VECTOR ( 'NONE', #46903, 1000.000000000000114 ) ;
#15826=DIRECTION ( 'NONE',  ( -0.9227826878668540234, -0.3853207896976547642, 0.000000000000000000 ) ) ;
#15829=VECTOR ( 'NONE', #20275, 1000.000000000000114 ) ;
#15830=DIRECTION ( 'NONE',  ( 0.9827303690289279636, 0.1850432970638682395, 0.000000000000000000 ) ) ;
#15833=DIRECTION ( 'NONE',  ( 0.9038112904824842087, -0.4279312458753000703, 0.000000000000000000 ) ) ;
#15836=LINE ( 'NONE', #4821, #8883 ) ;
#15837=ORIENTED_EDGE ( 'NONE', *, *, #38501, .F. ) ;
#15844=DIRECTION ( 'NONE',  ( -0.3853207896976547642, 0.9227826878668540234, 0.000000000000000000 ) ) ;
#15847=ORIENTED_EDGE ( 'NONE', *, *, #2059, .F. ) ;
#15858=DIRECTION ( 'NONE',  ( 0.4796670183876304283, -0.8774505977381978905, 0.000000000000000000 ) ) ;
#15862=EDGE_CURVE ( 'NONE', #1537, #13208, #35928, .T. ) ;
#15865=CYLINDRICAL_SURFACE ( 'NONE', #35341, 35.50000000000000711 ) ;
#15873=EDGE_CURVE ( 'NONE', #41996, #35358, #13423, .T. ) ;
#15885=ORIENTED_EDGE ( 'NONE', *, *, #44973, .T. ) ;
#15896=VERTEX_POINT ( 'NONE', #9748 ) ;
#15918=CARTESIAN_POINT ( 'NONE',  ( 23.49916127795269460, -121.5130826919798039, 2.500000000000000000 ) ) ;
#15923=EDGE_CURVE ( 'NONE', #30240, #37452, #6326, .T. ) ;
#15945=CARTESIAN_POINT ( 'NONE',  ( -1.459549131277904976, -119.6539995182286304, -2.500000000000000000 ) ) ;
#15948=EDGE_CURVE ( 'NONE', #29613, #43524, #16865, .T. ) ;
#15949=ORIENTED_EDGE ( 'NONE', *, *, #46189, .F. ) ;
#15950=VECTOR ( 'NONE', #26967, 1000.000000000000000 ) ;
#15951=CARTESIAN_POINT ( 'NONE',  ( -21.67772167707813935, -110.8034581014852762, -5.500000000000000000 ) ) ;
#15969=VECTOR ( 'NONE', #29079, 1000.000000000000114 ) ;
#15974=DIRECTION ( 'NONE',  ( 0.3311129884571281101, 0.9435911131814402886, 0.000000000000000000 ) ) ;
#15983=AXIS2_PLACEMENT_3D ( 'NONE', #44610, #44131, #14760 ) ;
#15987=LINE ( 'NONE', #35061, #1132 ) ;
#15999=DIRECTION ( 'NONE',  ( -0.000000000000000000, -0.000000000000000000, -1.000000000000000000 ) ) ;
#16022=DIRECTION ( 'NONE',  ( 0.5200609990132993854, 0.8541291221503275466, 0.000000000000000000 ) ) ;
#16030=VECTOR ( 'NONE', #14540, 1000.000000000000227 ) ;
#16037=ADVANCED_FACE ( 'NONE', ( #3108 ), #14640, .F. ) ;
#16041=PLANE ( 'NONE',  #21106 ) ;
#16054=ORIENTED_EDGE ( 'NONE', *, *, #8302, .T. ) ;
#16062=CARTESIAN_POINT ( 'NONE',  ( -21.67772167707813935, -110.8034581014852762, -2.500000000000000000 ) ) ;
#16064=DIRECTION ( 'NONE',  ( -0.3311129884571280546, -0.9435911131814402886, 0.000000000000000000 ) ) ;
#16065=LINE ( 'NONE', #8693, #45537 ) ;
#16071=VECTOR ( 'NONE', #36729, 1000.000000000000000 ) ;
#16072=AXIS2_PLACEMENT_3D ( 'NONE', #36829, #48100, #29499 ) ;
#16075=CARTESIAN_POINT ( 'NONE',  ( -3.961125083139900749, -143.2122702051246677, -5.500000000000000000 ) ) ;
#16091=EDGE_CURVE ( 'NONE', #43487, #33738, #18762, .T. ) ;
#16093=EDGE_LOOP ( 'NONE', ( #7427, #44573, #23801, #44014 ) ) ;
#16099=VERTEX_POINT ( 'NONE', #29794 ) ;
#16103=EDGE_CURVE ( 'NONE', #2158, #47361, #26377, .T. ) ;
#16119=VECTOR ( 'NONE', #37562, 1000.000000000000000 ) ;
#16165=ORIENTED_EDGE ( 'NONE', *, *, #35301, .T. ) ;
#16179=ORIENTED_EDGE ( 'NONE', *, *, #8334, .F. ) ;
#16196=LINE ( 'NONE', #38222, #16504 ) ;
#16201=CARTESIAN_POINT ( 'NONE',  ( 24.94940289813197509, -237.3777120880564553, 5.500000000000000000 ) ) ;
#16209=EDGE_CURVE ( 'NONE', #20931, #28111, #16334, .T. ) ;
#16235=FACE_OUTER_BOUND ( 'NONE', #30110, .T. ) ;
#16245=ORIENTED_EDGE ( 'NONE', *, *, #28069, .T. ) ;
#16256=EDGE_CURVE ( 'NONE', #26232, #37461, #23428, .T. ) ;
#16266=ORIENTED_EDGE ( 'NONE', *, *, #7662, .F. ) ;
#16282=PLANE ( 'NONE',  #44144 ) ;
#16290=AXIS2_PLACEMENT_3D ( 'NONE', #39916, #20577, #9325 ) ;
#16296=DIRECTION ( 'NONE',  ( 0.6862798483830534479, 0.7273375899149810975, 0.000000000000000000 ) ) ;
#16302=DIRECTION ( 'NONE',  ( 0.5200609990132993854, 0.8541291221503275466, -0.000000000000000000 ) ) ;
#16307=FACE_OUTER_BOUND ( 'NONE', #29742, .T. ) ;
#16334=LINE ( 'NONE', #3931, #1888 ) ;
#16341=LINE ( 'NONE', #31780, #17258 ) ;
#16349=ORIENTED_EDGE ( 'NONE', *, *, #7293, .F. ) ;
#16361=CARTESIAN_POINT ( 'NONE',  ( 23.11608002360578240, -124.4885236261218182, 5.500000000000000000 ) ) ;
#16363=CARTESIAN_POINT ( 'NONE',  ( 16.84844760790522855, -103.5491698323862124, 5.500000000000000000 ) ) ;
#16376=CARTESIAN_POINT ( 'NONE',  ( 1.233757462863572574, -119.1468631277289347, 2.500000000000000000 ) ) ;
#16389=ORIENTED_EDGE ( 'NONE', *, *, #7828, .F. ) ;
#16413=EDGE_LOOP ( 'NONE', ( #23843, #19099, #32074, #12082 ) ) ;
#16436=ADVANCED_FACE ( 'NONE', ( #22170 ), #7236, .F. ) ;
#16457=ORIENTED_EDGE ( 'NONE', *, *, #7828, .T. ) ;
#16458=ADVANCED_FACE ( 'NONE', ( #7719 ), #33429, .T. ) ;
#16463=ADVANCED_FACE ( 'NONE', ( #44444 ), #10430, .F. ) ;
#16465=DIRECTION ( 'NONE',  ( -0.9918136447140104561, 0.1276937514489679681, 0.000000000000000000 ) ) ;
#16469=EDGE_LOOP ( 'NONE', ( #45226, #47442, #35795, #181 ) ) ;
#16470=CARTESIAN_POINT ( 'NONE',  ( -12.50000000000000000, -107.5000000000000000, -2.500000000000000000 ) ) ;
#16479=CARTESIAN_POINT ( 'NONE',  ( 24.95699195200416654, -110.9640411295978595, 5.500000000000000000 ) ) ;
#16504=VECTOR ( 'NONE', #23287, 1000.000000000000000 ) ;
#16569=AXIS2_PLACEMENT_3D ( 'NONE', #2034, #9584, #6177 ) ;
#16575=VECTOR ( 'NONE', #6256, 1000.000000000000000 ) ;
#16584=DIRECTION ( 'NONE',  ( 0.9038112904824842087, -0.4279312458753000703, 0.000000000000000000 ) ) ;
#16612=ORIENTED_EDGE ( 'NONE', *, *, #28874, .T. ) ;
#16615=SURFACE_STYLE_USAGE ( .BOTH. , #20042 ) ;
#16619=ADVANCED_FACE ( 'NONE', ( #15327 ), #16282, .F. ) ;
#16630=ORIENTED_EDGE ( 'NONE', *, *, #46052, .F. ) ;
#16641=VERTEX_POINT ( 'NONE', #22888 ) ;
#16651=CYLINDRICAL_SURFACE ( 'NONE', #28951, 30.50000000000000000 ) ;
#16664=FACE_OUTER_BOUND ( 'NONE', #45405, .T. ) ;
#16669=CARTESIAN_POINT ( 'NONE',  ( -14.25258209288423750, -138.6845900058201551, 2.500000000000000000 ) ) ;
#16677=EDGE_CURVE ( 'NONE', #19426, #3571, #45400, .T. ) ;
#16694=DIRECTION ( 'NONE',  ( -1.000000000000000000, 0.000000000000000000, 0.000000000000000000 ) ) ;
#16718=VECTOR ( 'NONE', #6484, 1000.000000000000000 ) ;
#16732=ORIENTED_EDGE ( 'NONE', *, *, #35252, .T. ) ;
#16743=VERTEX_POINT ( 'NONE', #13820 ) ;
#16750=VERTEX_POINT ( 'NONE', #32180 ) ;
#16756=VERTEX_POINT ( 'NONE', #35837 ) ;
#16759=VECTOR ( 'NONE', #5605, 1000.000000000000114 ) ;
#16771=LINE ( 'NONE', #13336, #3014 ) ;
#16806=AXIS2_PLACEMENT_3D ( 'NONE', #34400, #12175, #4343 ) ;
#16808=DIRECTION ( 'NONE',  ( -0.9781476007338069101, 0.2079116908177532363, 0.000000000000000000 ) ) ;
#16816=ADVANCED_FACE ( 'NONE', ( #1834 ), #31715, .F. ) ;
#16828=EDGE_LOOP ( 'NONE', ( #8324, #40526, #27400, #44124 ) ) ;
#16835=LINE ( 'NONE', #32015, #4406 ) ;
#16840=AXIS2_PLACEMENT_3D ( 'NONE', #46166, #38836, #24132 ) ;
#16865=LINE ( 'NONE', #13906, #16759 ) ;
#16869=EDGE_CURVE ( 'NONE', #36710, #15673, #37039, .T. ) ;
#16870=EDGE_LOOP ( 'NONE', ( #36142, #8313, #6337, #38389 ) ) ;
#16875=DIRECTION ( 'NONE',  ( -0.3311129884571281101, -0.9435911131814402886, 0.000000000000000000 ) ) ;
#16882=EDGE_LOOP ( 'NONE', ( #23267, #27410, #32123, #11532 ) ) ;
#16906=CIRCLE ( 'NONE', #37196, 35.50000000000000711 ) ;
#16907=LINE ( 'NONE', #43092, #5549 ) ;
#16910=PLANE ( 'NONE',  #9108 ) ;
#16911=CARTESIAN_POINT ( 'NONE',  ( -23.42219527698293646, -121.9106984081423803, 2.500000000000000000 ) ) ;
#16913=VECTOR ( 'NONE', #11074, 1000.000000000000000 ) ;
#16918=VECTOR ( 'NONE', #36979, 1000.000000000000000 ) ;
#16919=PLANE ( 'NONE',  #3805 ) ;
#16923=EDGE_CURVE ( 'NONE', #17280, #32168, #44389, .T. ) ;
#16927=CARTESIAN_POINT ( 'NONE',  ( 0.000000000000000000, -120.0000000000000000, 2.500000000000000000 ) ) ;
#16929=EDGE_CURVE ( 'NONE', #47410, #31423, #48295, .T. ) ;
#16931=ORIENTED_EDGE ( 'NONE', *, *, #41221, .F. ) ;
#16944=DIRECTION ( 'NONE',  ( 1.000000000000000000, 0.000000000000000000, -0.000000000000000000 ) ) ;
#16947=DIRECTION ( 'NONE',  ( -0.000000000000000000, -0.000000000000000000, 1.000000000000000000 ) ) ;
#16948=ADVANCED_FACE ( 'NONE', ( #29935 ), #44872, .F. ) ;
#16955=DIRECTION ( 'NONE',  ( -0.000000000000000000, -0.000000000000000000, -1.000000000000000000 ) ) ;
#16956=VERTEX_POINT ( 'NONE', #21383 ) ;
#16980=DIRECTION ( 'NONE',  ( 0.8774505977381971134, 0.4796670183876317051, -0.000000000000000000 ) ) ;
#16986=VERTEX_POINT ( 'NONE', #31161 ) ;
#16990=DIRECTION ( 'NONE',  ( -0.7950889364178781449, 0.6064928550163533050, 0.000000000000000000 ) ) ;
#17001=EDGE_CURVE ( 'NONE', #43248, #18614, #567, .T. ) ;
#17026=DIRECTION ( 'NONE',  ( 0.9135454576426059736, -0.4067366430757887730, 0.000000000000000000 ) ) ;
#17029=CARTESIAN_POINT ( 'NONE',  ( -12.50000000000000000, -107.5000000000000000, 2.500000000000000000 ) ) ;
#17034=ORIENTED_EDGE ( 'NONE', *, *, #43357, .F. ) ;
#17038=VERTEX_POINT ( 'NONE', #34813 ) ;
#17045=EDGE_LOOP ( 'NONE', ( #23014, #14468, #25470, #43197 ) ) ;
#17068=EDGE_CURVE ( 'NONE', #36858, #6148, #23317, .T. ) ;
#17071=EDGE_CURVE ( 'NONE', #7858, #4059, #26751, .T. ) ;
#17073=EDGE_CURVE ( 'NONE', #37535, #13263, #8616, .T. ) ;
#17090=DIRECTION ( 'NONE',  ( -0.6516173805718079581, 0.7585478161175706058, 0.000000000000000000 ) ) ;
#17095=ORIENTED_EDGE ( 'NONE', *, *, #43811, .F. ) ;
#17101=VECTOR ( 'NONE', #17796, 1000.000000000000114 ) ;
#17111=VERTEX_POINT ( 'NONE', #5685 ) ;
#17112=EDGE_CURVE ( 'NONE', #28620, #29568, #31654, .T. ) ;
#17135=AXIS2_PLACEMENT_3D ( 'NONE', #896, #15844, #10967 ) ;
#17137=DIRECTION ( 'NONE',  ( 1.000000000000000000, 0.000000000000000000, 0.000000000000000000 ) ) ;
#17140=FACE_OUTER_BOUND ( 'NONE', #7910, .T. ) ;
#17151=CYLINDRICAL_SURFACE ( 'NONE', #14327, 35.50000000000000711 ) ;
#17155=VECTOR ( 'NONE', #10827, 1000.000000000000000 ) ;
#17163=CARTESIAN_POINT ( 'NONE',  ( 21.85433023846371370, -135.0628101570779620, 5.500000000000000000 ) ) ;
#17177=VERTEX_POINT ( 'NONE', #28436 ) ;
#17179=EDGE_CURVE ( 'NONE', #4059, #14947, #42896, .T. ) ;
#17188=LINE ( 'NONE', #40213, #4800 ) ;
#17196=CARTESIAN_POINT ( 'NONE',  ( 26.47460221209471598, -121.8961639463267090, 5.500000000000000000 ) ) ;
#17197=LINE ( 'NONE', #23170, #44148 ) ;
#17199=DIRECTION ( 'NONE',  ( -0.000000000000000000, -0.000000000000000000, -1.000000000000000000 ) ) ;
#17200=ORIENTED_EDGE ( 'NONE', *, *, #21251, .T. ) ;
#17202=EDGE_LOOP ( 'NONE', ( #19674, #25042, #4358, #15131 ) ) ;
#17212=ORIENTED_EDGE ( 'NONE', *, *, #12001, .T. ) ;
#17213=ADVANCED_FACE ( 'NONE', ( #39715 ), #17404, .F. ) ;
#17218=DIRECTION ( 'NONE',  ( -0.7273375899149793211, 0.6862798483830554463, 0.000000000000000000 ) ) ;
#17252=PLANE ( 'NONE',  #37013 ) ;
#17258=VECTOR ( 'NONE', #31283, 1000.000000000000114 ) ;
#17271=EDGE_CURVE ( 'NONE', #16099, #29948, #24995, .T. ) ;
#17280=VERTEX_POINT ( 'NONE', #36496 ) ;
#17292=VERTEX_POINT ( 'NONE', #43841 ) ;
#17297=FACE_BOUND ( 'NONE', #35731, .T. ) ;
#17320=PRESENTATION_STYLE_ASSIGNMENT (( #16615 ) ) ;
#17327=AXIS2_PLACEMENT_3D ( 'NONE', #12553, #27491, #12796 ) ;
#17333=VECTOR ( 'NONE', #37064, 1000.000000000000000 ) ;
#17344=EDGE_CURVE ( 'NONE', #41379, #21334, #10803, .T. ) ;
#17345=ORIENTED_EDGE ( 'NONE', *, *, #16256, .T. ) ;
#17351=DIRECTION ( 'NONE',  ( -0.02332147558787674158, -0.9997280174009349762, 0.000000000000000000 ) ) ;
#17354=DIRECTION ( 'NONE',  ( 1.000000000000000000, 0.000000000000000000, 0.000000000000000000 ) ) ;
#17389=VECTOR ( 'NONE', #542, 1000.000000000000000 ) ;
#17404=PLANE ( 'NONE',  #25441 ) ;
#17436=DIRECTION ( 'NONE',  ( -0.000000000000000000, -0.000000000000000000, -1.000000000000000000 ) ) ;
#17472=EDGE_CURVE ( 'NONE', #37298, #12589, #41880, .T. ) ;
#17483=CARTESIAN_POINT ( 'NONE',  ( 2.117611129180199558, -93.54218975225703048, 5.500000000000000000 ) ) ;
#17496=EDGE_LOOP ( 'NONE', ( #16630, #22279, #35561, #34261 ) ) ;
#17520=VECTOR ( 'NONE', #23188, 1000.000000000000114 ) ;
#17545=FACE_BOUND ( 'NONE', #48162, .T. ) ;
#17546=LINE ( 'NONE', #33208, #37815 ) ;
#17550=CARTESIAN_POINT ( 'NONE',  ( -1.499592026101402853, -119.9650177866181764, -2.500000000000000000 ) ) ;
#17554=VERTEX_POINT ( 'NONE', #9062 ) ;
#17602=ADVANCED_FACE ( 'NONE', ( #46028 ), #9525, .F. ) ;
#17606=EDGE_CURVE ( 'NONE', #4059, #45971, #20801, .T. ) ;
#17612=VERTEX_POINT ( 'NONE', #24716 ) ;
#17613=ADVANCED_FACE ( 'NONE', ( #1478 ), #20073, .T. ) ;
#17627=LINE ( 'NONE', #21292, #26439 ) ;
#17639=AXIS2_PLACEMENT_3D ( 'NONE', #12323, #16465, #38758 ) ;
#17642=EDGE_CURVE ( 'NONE', #38166, #28952, #38464, .T. ) ;
#17649=CARTESIAN_POINT ( 'NONE',  ( -14.87942725330654348, -141.9795960975983178, -5.500000000000000000 ) ) ;
#17666=EDGE_LOOP ( 'NONE', ( #33980, #13218, #19856, #11600 ) ) ;
#17675=DIRECTION ( 'NONE',  ( -0.000000000000000000, -0.000000000000000000, -1.000000000000000000 ) ) ;
#17680=CIRCLE ( 'NONE', #7552, 35.50000000000000711 ) ;
#17689=EDGE_CURVE ( 'NONE', #24295, #34363, #10016, .T. ) ;
#17714=EDGE_LOOP ( 'NONE', ( #44641, #25966, #47871, #46033 ) ) ;
#17752=LINE ( 'NONE', #32677, #38100 ) ;
#17790=CARTESIAN_POINT ( 'NONE',  ( -26.53422223201112828, -120.6595836127786043, 5.500000000000000000 ) ) ;
#17795=ORIENTED_EDGE ( 'NONE', *, *, #23652, .F. ) ;
#17796=DIRECTION ( 'NONE',  ( 0.3853207896976533209, -0.9227826878668545785, 0.000000000000000000 ) ) ;
#17802=EDGE_CURVE ( 'NONE', #28317, #45238, #18793, .T. ) ;
#17805=CARTESIAN_POINT ( 'NONE',  ( -24.50849501662245444, -109.8101191361138831, 2.500000000000000000 ) ) ;
#17806=CARTESIAN_POINT ( 'NONE',  ( 2.047646702416564768, -96.54137380445985173, 5.500000000000000000 ) ) ;
#17808=CARTESIAN_POINT ( 'NONE',  ( 16.84844760790522855, -103.5491698323862124, 5.500000000000000000 ) ) ;
#17837=ORIENTED_EDGE ( 'NONE', *, *, #26188, .F. ) ;
#17840=ADVANCED_FACE ( 'NONE', ( #454 ), #15865, .T. ) ;
#17883=CARTESIAN_POINT ( 'NONE',  ( -23.97194136764370498, -131.3950000906648938, 5.500000000000000000 ) ) ;
#17888=AXIS2_PLACEMENT_3D ( 'NONE', #11691, #4111, #4587 ) ;
#17895=LINE ( 'NONE', #13279, #29260 ) ;
#17897=ADVANCED_FACE ( 'NONE', ( #5827 ), #4848, .F. ) ;
#17904=ORIENTED_EDGE ( 'NONE', *, *, #44548, .F. ) ;
#17906=DIRECTION ( 'NONE',  ( 0.2306669878475637314, 0.9730327541852493711, 0.000000000000000000 ) ) ;
#17907=CARTESIAN_POINT ( 'NONE',  ( -26.29030328629083968, -123.6496510949466341, -5.500000000000000000 ) ) ;
#17916=CARTESIAN_POINT ( 'NONE',  ( -26.41226275915097332, -122.1546173538626761, 2.500000000000000000 ) ) ;
#17955=EDGE_LOOP ( 'NONE', ( #20958, #80, #44289, #32679 ) ) ;
#17961=CARTESIAN_POINT ( 'NONE',  ( 5.822613034544236399, -142.8165987265839760, 2.500000000000000000 ) ) ;
#17964=CARTESIAN_POINT ( 'NONE',  ( 11.41210121379328335, -99.40233154247455616, 5.500000000000000000 ) ) ;
#17965=LINE ( 'NONE', #32899, #4946 ) ;
#17969=EDGE_CURVE ( 'NONE', #21334, #24269, #2150, .T. ) ;
#17971=VERTEX_POINT ( 'NONE', #39343 ) ;
#17981=DIRECTION ( 'NONE',  ( -0.000000000000000000, -0.000000000000000000, -1.000000000000000000 ) ) ;
#17982=LINE ( 'NONE', #21676, #33796 ) ;
#17987=EDGE_CURVE ( 'NONE', #4822, #12549, #32017, .T. ) ;
#17997=DIRECTION ( 'NONE',  ( 0.3311129884571281101, 0.9435911131814402886, -0.000000000000000000 ) ) ;
#17998=CIRCLE ( 'NONE', #34422, 35.50000000000000711 ) ;
#18009=DIRECTION ( 'NONE',  ( 0.4279312458752991266, 0.9038112904824847638, 0.000000000000000000 ) ) ;
#18018=FACE_BOUND ( 'NONE', #32295, .T. ) ;
#18030=AXIS2_PLACEMENT_3D ( 'NONE', #31429, #20377, #38772 ) ;
#18037=VECTOR ( 'NONE', #26968, 1000.000000000000000 ) ;
#18039=FACE_OUTER_BOUND ( 'NONE', #35676, .T. ) ;
#18056=PLANE ( 'NONE',  #40578 ) ;
#18058=AXIS2_PLACEMENT_3D ( 'NONE', #10197, #43017, #32478 ) ;
#18064=DIRECTION ( 'NONE',  ( 0.1850432970638667407, -0.9827303690289282967, 0.000000000000000000 ) ) ;
#18080=DIRECTION ( 'NONE',  ( 0.9038112904824853189, -0.4279312458752977388, 0.000000000000000000 ) ) ;
#18083=VERTEX_POINT ( 'NONE', #7442 ) ;
#18086=DIRECTION ( 'NONE',  ( -0.8225049752423776450, -0.5687579148473765889, 0.000000000000000000 ) ) ;
#18088=DIRECTION ( 'NONE',  ( -0.5200609990132993854, -0.8541291221503274356, 0.000000000000000000 ) ) ;
#18102=AXIS2_PLACEMENT_3D ( 'NONE', #40559, #41294, #11445 ) ;
#18106=VECTOR ( 'NONE', #45974, 1000.000000000000000 ) ;
#18108=LINE ( 'NONE', #33046, #32351 ) ;
#18121=CARTESIAN_POINT ( 'NONE',  ( -10.43921258969510824, -98.89258801967538659, 5.500000000000000000 ) ) ;
#18144=CARTESIAN_POINT ( 'NONE',  ( 12.50000000000000000, -132.5000000000000000, -2.500000000000000000 ) ) ;
#18158=AXIS2_PLACEMENT_3D ( 'NONE', #29186, #20896, #47072 ) ;
#18159=ORIENTED_EDGE ( 'NONE', *, *, #40056, .T. ) ;
#18162=ORIENTED_EDGE ( 'NONE', *, *, #46716, .T. ) ;
#18169=EDGE_CURVE ( 'NONE', #19505, #24549, #19400, .T. ) ;
#18186=ORIENTED_EDGE ( 'NONE', *, *, #12187, .F. ) ;
#18188=CARTESIAN_POINT ( 'NONE',  ( 0.4301293587033142574, -121.4370068666438556, -2.500000000000000000 ) ) ;
#18200=LINE ( 'NONE', #3523, #25410 ) ;
#18207=DIRECTION ( 'NONE',  ( 0.9918136447140104561, -0.1276937514489679681, 0.000000000000000000 ) ) ;
#18216=LINE ( 'NONE', #9737, #38056 ) ;
#18218=DIRECTION ( 'NONE',  ( 1.000000000000000000, 0.000000000000000000, 0.000000000000000000 ) ) ;
#18256=FACE_BOUND ( 'NONE', #10232, .T. ) ;
#18257=EDGE_LOOP ( 'NONE', ( #38121, #44021, #40144, #28603 ) ) ;
#18268=CARTESIAN_POINT ( 'NONE',  ( 26.47460221209471598, -121.8961639463267090, 5.500000000000000000 ) ) ;
#18306=DIRECTION ( 'NONE',  ( -0.3853207896976547642, 0.9227826878668540234, 0.000000000000000000 ) ) ;
#18309=EDGE_LOOP ( 'NONE', ( #10031, #21853, #37151, #5346 ) ) ;
#18327=VERTEX_POINT ( 'NONE', #27251 ) ;
#18328=CARTESIAN_POINT ( 'NONE',  ( 30.50000000000000000, -120.0000000000000000, 2.500000000000000000 ) ) ;
#18330=DIRECTION ( 'NONE',  ( -0.9918136447140101231, 0.1276937514489694114, 0.000000000000000000 ) ) ;
#18373=ORIENTED_EDGE ( 'NONE', *, *, #29855, .T. ) ;
#18389=DIRECTION ( 'NONE',  ( -0.9435911131814398445, 0.3311129884571295534, 0.000000000000000000 ) ) ;
#18394=LINE ( 'NONE', #33326, #45165 ) ;
#18414=PLANE ( 'NONE',  #30054 ) ;
#18415=CARTESIAN_POINT ( 'NONE',  ( -8.826826895187510402, -94.96827758698185562, 5.500000000000000000 ) ) ;
#18418=VECTOR ( 'NONE', #5856, 1000.000000000000000 ) ;
#18422=CARTESIAN_POINT ( 'NONE',  ( 26.47460221209471598, -121.8961639463267090, 5.500000000000000000 ) ) ;
#18437=DIRECTION ( 'NONE',  ( 0.000000000000000000, 0.000000000000000000, 1.000000000000000000 ) ) ;
#18439=FACE_OUTER_BOUND ( 'NONE', #31399, .T. ) ;
#18447=DIRECTION ( 'NONE',  ( -0.02332147558787930897, -0.9997280174009348652, 0.000000000000000000 ) ) ;
#18452=ORIENTED_EDGE ( 'NONE', *, *, #7662, .T. ) ;
#18464=EDGE_CURVE ( 'NONE', #11806, #28861, #30490, .T. ) ;
#18465=CARTESIAN_POINT ( 'NONE',  ( -0.4301293587032979371, -118.5629931333561871, 2.500000000000000000 ) ) ;
#18467=DIRECTION ( 'NONE',  ( -0.000000000000000000, -0.000000000000000000, 1.000000000000000000 ) ) ;
#18470=ORIENTED_EDGE ( 'NONE', *, *, #44597, .F. ) ;
#18476=DIRECTION ( 'NONE',  ( 0.02332147558787931590, 0.9997280174009348652, 0.000000000000000000 ) ) ;
#18493=VERTEX_POINT ( 'NONE', #25485 ) ;
#18498=CARTESIAN_POINT ( 'NONE',  ( -15.44521549751111422, -137.7748507232956001, 5.500000000000000000 ) ) ;
#18507=DIRECTION ( 'NONE',  ( 0.02332147558787931590, 0.9997280174009348652, 0.000000000000000000 ) ) ;
#18519=CARTESIAN_POINT ( 'NONE',  ( 23.41451323550360186, -132.5004227906269989, 5.500000000000000000 ) ) ;
#18523=EDGE_CURVE ( 'NONE', #13979, #37298, #11048, .T. ) ;
#18536=CARTESIAN_POINT ( 'NONE',  ( -1.384174031800281979, -120.5779811845464735, -2.500000000000000000 ) ) ;
#18554=DIRECTION ( 'NONE',  ( 0.9135454576426059736, -0.4067366430757887730, 0.000000000000000000 ) ) ;
#18561=EDGE_CURVE ( 'NONE', #36710, #34363, #14965, .T. ) ;
#18568=DIRECTION ( 'NONE',  ( -0.000000000000000000, -0.000000000000000000, 1.000000000000000000 ) ) ;
#18587=FACE_OUTER_BOUND ( 'NONE', #43971, .T. ) ;
#18594=LINE ( 'NONE', #14924, #30129 ) ;
#18614=VERTEX_POINT ( 'NONE', #7853 ) ;
#18620=ORIENTED_EDGE ( 'NONE', *, *, #35671, .T. ) ;
#18658=ORIENTED_EDGE ( 'NONE', *, *, #13389, .T. ) ;
#18661=VERTEX_POINT ( 'NONE', #34508 ) ;
#18685=ORIENTED_EDGE ( 'NONE', *, *, #27575, .T. ) ;
#18705=ADVANCED_FACE ( 'NONE', ( #18857 ), #41630, .T. ) ;
#18706=DIRECTION ( 'NONE',  ( -0.9435911131814395114, 0.3311129884571304971, 0.000000000000000000 ) ) ;
#18712=EDGE_CURVE ( 'NONE', #35445, #32049, #8096, .T. ) ;
#18723=VECTOR ( 'NONE', #41499, 1000.000000000000000 ) ;
#18728=DIRECTION ( 'NONE',  ( -0.000000000000000000, -0.000000000000000000, -1.000000000000000000 ) ) ;
#18731=( GEOMETRIC_REPRESENTATION_CONTEXT ( 3 ) GLOBAL_UNCERTAINTY_ASSIGNED_CONTEXT ( ( #34479 ) ) GLOBAL_UNIT_ASSIGNED_CONTEXT ( ( #37118, #11183, #37847 ) ) REPRESENTATION_CONTEXT ( 'NONE', 'WORKASPACE' ) );
#18745=LINE ( 'NONE', #18519, #26035 ) ;
#18757=DIRECTION ( 'NONE',  ( 0.5687579148473765889, -0.8225049752423776450, 0.000000000000000000 ) ) ;
#18761=PLANE ( 'NONE',  #9892 ) ;
#18762=LINE ( 'NONE', #14146, #324 ) ;
#18766=CARTESIAN_POINT ( 'NONE',  ( -16.06301359042743115, -102.7814171781257357, 5.500000000000000000 ) ) ;
#18771=AXIS2_PLACEMENT_3D ( 'NONE', #19408, #22611, #41700 ) ;
#18773=EDGE_LOOP ( 'NONE', ( #7519, #4997, #21032, #15652 ) ) ;
#18775=PLANE ( 'NONE',  #24161 ) ;
#18778=EDGE_CURVE ( 'NONE', #32168, #13208, #17998, .T. ) ;
#18783=DIRECTION ( 'NONE',  ( -0.8541291221503266584, 0.5200609990133008287, 0.000000000000000000 ) ) ;
#18785=DIRECTION ( 'NONE',  ( -0.000000000000000000, -0.000000000000000000, -1.000000000000000000 ) ) ;
#18786=EDGE_LOOP ( 'NONE', ( #26157, #16457, #41155, #16054 ) ) ;
#18793=LINE ( 'NONE', #33973, #46292 ) ;
#18799=VECTOR ( 'NONE', #43333, 1000.000000000000000 ) ;
#18805=EDGE_LOOP ( 'NONE', ( #37370, #12418, #46964, #44726 ) ) ;
#18821=FACE_OUTER_BOUND ( 'NONE', #31449, .T. ) ;
#18827=EDGE_CURVE ( 'NONE', #28062, #30774, #20080, .T. ) ;
#18830=DIRECTION ( 'NONE',  ( -0.5000000000000039968, 0.8660254037844363761, 0.000000000000000000 ) ) ;
#18844=ADVANCED_FACE ( 'NONE', ( #35734 ), #16651, .F. ) ;
#18857=FACE_OUTER_BOUND ( 'NONE', #27662, .T. ) ;
#18863=CARTESIAN_POINT ( 'NONE',  ( -22.53294031248082163, -134.0273518838794757, 5.500000000000000000 ) ) ;
#18872=DIRECTION ( 'NONE',  ( 0.000000000000000000, 1.000000000000000000, 0.000000000000000000 ) ) ;
#18874=LINE ( 'NONE', #19365, #19988 ) ;
#18896=VECTOR ( 'NONE', #38759, 1000.000000000000227 ) ;
#18897=VECTOR ( 'NONE', #19567, 1000.000000000000114 ) ;
#18911=LINE ( 'NONE', #571, #39799 ) ;
#18913=EDGE_CURVE ( 'NONE', #47361, #39725, #47691, .T. ) ;
#18926=LINE ( 'NONE', #37789, #33645 ) ;
#18930=CARTESIAN_POINT ( 'NONE',  ( 22.94323693612312454, -114.6983135802921083, -2.500000000000000000 ) ) ;
#18947=EDGE_CURVE ( 'NONE', #8139, #26232, #6598, .T. ) ;
#18966=ORIENTED_EDGE ( 'NONE', *, *, #38974, .F. ) ;
#18971=LINE ( 'NONE', #33907, #15779 ) ;
#18975=VERTEX_POINT ( 'NONE', #18328 ) ;
#18987=DIRECTION ( 'NONE',  ( -0.9918136447140100120, 0.1276937514489704939, 0.000000000000000000 ) ) ;
#18991=PLANE ( 'NONE',  #18102 ) ;
#19033=LINE ( 'NONE', #22711, #13401 ) ;
#19069=FACE_OUTER_BOUND ( 'NONE', #40660, .T. ) ;
#19070=DIRECTION ( 'NONE',  ( -0.02332147558787823344, -0.9997280174009349762, 0.000000000000000000 ) ) ;
#19071=DIRECTION ( 'NONE',  ( 0.9038112904824853189, -0.4279312458752977388, 0.000000000000000000 ) ) ;
#19099=ORIENTED_EDGE ( 'NONE', *, *, #10394, .T. ) ;
#19103=ADVANCED_FACE ( 'NONE', ( #7566 ), #4393, .F. ) ;
#19112=LINE ( 'NONE', #748, #37332 ) ;
#19113=VERTEX_POINT ( 'NONE', #15157 ) ;
#19122=CARTESIAN_POINT ( 'NONE',  ( -4.653126046682595884, -146.1313684676804314, 5.500000000000000000 ) ) ;
#19154=ORIENTED_EDGE ( 'NONE', *, *, #6211, .F. ) ;
#19177=EDGE_CURVE ( 'NONE', #3188, #12549, #13170, .T. ) ;
#19187=LINE ( 'NONE', #342, #46314 ) ;
#19190=DIRECTION ( 'NONE',  ( -0.9038112904824853189, 0.4279312458752976833, 0.000000000000000000 ) ) ;
#19240=CARTESIAN_POINT ( 'NONE',  ( 0.4966694826857007139, -118.5846133302278247, -2.500000000000000000 ) ) ;
#19286=EDGE_LOOP ( 'NONE', ( #36252, #5324, #9898, #28303 ) ) ;
#19306=CARTESIAN_POINT ( 'NONE',  ( 1.459549131277868561, -120.3460004817713411, 2.500000000000000000 ) ) ;
#19312=LINE ( 'NONE', #39074, #24625 ) ;
#19320=EDGE_CURVE ( 'NONE', #41947, #28440, #40336, .T. ) ;
#19337=ORIENTED_EDGE ( 'NONE', *, *, #35614, .F. ) ;
#19344=ORIENTED_EDGE ( 'NONE', *, *, #22828, .T. ) ;
#19353=CARTESIAN_POINT ( 'NONE',  ( -21.33958957442910886, -129.9559990355020034, 5.500000000000000000 ) ) ;
#19365=CARTESIAN_POINT ( 'NONE',  ( 12.50000000000000000, -107.5000000000000000, 2.500000000000000000 ) ) ;
#19373=AXIS2_PLACEMENT_3D ( 'NONE', #45408, #26814, #18507 ) ;
#19374=ORIENTED_EDGE ( 'NONE', *, *, #11932, .F. ) ;
#19375=EDGE_CURVE ( 'NONE', #27608, #27838, #36150, .T. ) ;
#19382=ADVANCED_FACE ( 'NONE', ( #10456 ), #10938, .F. ) ;
#19385=CARTESIAN_POINT ( 'NONE',  ( -24.50849501662245800, -109.8101191361138831, 5.500000000000000000 ) ) ;
#19391=DIRECTION ( 'NONE',  ( -0.8225049752423776450, -0.5687579148473765889, 0.000000000000000000 ) ) ;
#19400=LINE ( 'NONE', #45860, #7773 ) ;
#19406=ORIENTED_EDGE ( 'NONE', *, *, #26188, .T. ) ;
#19408=CARTESIAN_POINT ( 'NONE',  ( -16.06301359042743115, -102.7814171781257357, 5.500000000000000000 ) ) ;
#19411=DIRECTION ( 'NONE',  ( 0.000000000000000000, -0.000000000000000000, 1.000000000000000000 ) ) ;
#19413=CARTESIAN_POINT ( 'NONE',  ( -11.59517495878806947, -96.12423995607481686, 2.500000000000000000 ) ) ;
#19421=MANIFOLD_SOLID_BREP ( 'Revolve1', #30197 ) ;
#19426=VERTEX_POINT ( 'NONE', #41524 ) ;
#19440=CARTESIAN_POINT ( 'NONE',  ( -12.50000000000000000, -132.5000000000000000, 2.500000000000000000 ) ) ;
#19458=DIRECTION ( 'NONE',  ( -0.9227826878668545785, -0.3853207896976533209, 0.000000000000000000 ) ) ;
#19469=DIRECTION ( 'NONE',  ( -0.8090169943749426773, -0.5877852522924797984, 0.000000000000000000 ) ) ;
#19471=VERTEX_POINT ( 'NONE', #30503 ) ;
#19473=FACE_OUTER_BOUND ( 'NONE', #3731, .T. ) ;
#19482=EDGE_CURVE ( 'NONE', #40068, #47873, #4333, .T. ) ;
#19505=VERTEX_POINT ( 'NONE', #31485 ) ;
#19516=DIRECTION ( 'NONE',  ( -0.9918136447140101231, 0.1276937514489694114, 0.000000000000000000 ) ) ;
#19518=VECTOR ( 'NONE', #31216, 1000.000000000000000 ) ;
#19528=VECTOR ( 'NONE', #27261, 1000.000000000000000 ) ;
#19536=EDGE_CURVE ( 'NONE', #47237, #7713, #8467, .T. ) ;
#19545=DIRECTION ( 'NONE',  ( 1.000000000000000000, 0.000000000000000000, 0.000000000000000000 ) ) ;
#19567=DIRECTION ( 'NONE',  ( -0.6862798483830534479, -0.7273375899149810975, 0.000000000000000000 ) ) ;
#19570=VERTEX_POINT ( 'NONE', #20690 ) ;
#19590=LINE ( 'NONE', #15951, #23133 ) ;
#19612=SHAPE_DEFINITION_REPRESENTATION ( #12414, #29385 ) ;
#19623=CARTESIAN_POINT ( 'NONE',  ( -19.90058851926621131, -132.5883508287165853, 5.500000000000000000 ) ) ;
#19647=ORIENTED_EDGE ( 'NONE', *, *, #26251, .T. ) ;
#19668=AXIS2_PLACEMENT_3D ( 'NONE', #25229, #6411, #40191 ) ;
#19674=ORIENTED_EDGE ( 'NONE', *, *, #16256, .F. ) ;
#19688=CARTESIAN_POINT ( 'NONE',  ( 9.984461079971730157, -95.40710393340120277, -5.500000000000000000 ) ) ;
#19714=DIRECTION ( 'NONE',  ( -0.9730327541852497042, 0.2306669878475623159, 0.000000000000000000 ) ) ;
#19725=VERTEX_POINT ( 'NONE', #35539 ) ;
#19731=CARTESIAN_POINT ( 'NONE',  ( -14.87942725330654348, -141.9795960975983178, 5.500000000000000000 ) ) ;
#19772=VECTOR ( 'NONE', #31735, 1000.000000000000000 ) ;
#19793=CARTESIAN_POINT ( 'NONE',  ( -0.9515373497862389396, -96.47140937769621871, 5.500000000000000000 ) ) ;
#19795=LINE ( 'NONE', #28124, #47198 ) ;
#19805=EDGE_CURVE ( 'NONE', #44934, #34735, #38980, .T. ) ;
#19812=VECTOR ( 'NONE', #23759, 1000.000000000000000 ) ;
#19837=CARTESIAN_POINT ( 'NONE',  ( -18.12185313557660038, -104.9634299478706794, 5.500000000000000000 ) ) ;
#19856=ORIENTED_EDGE ( 'NONE', *, *, #18712, .T. ) ;
#19863=DIRECTION ( 'NONE',  ( 0.9435911131814402886, -0.3311129884571281101, 0.000000000000000000 ) ) ;
#19870=VECTOR ( 'NONE', #4052, 1000.000000000000000 ) ;
#19877=ADVANCED_FACE ( 'NONE', ( #43603 ), #36723, .F. ) ;
#19897=EDGE_CURVE ( 'NONE', #18083, #10970, #24766, .T. ) ;
#19898=LINE ( 'NONE', #31674, #19528 ) ;
#19905=DIRECTION ( 'NONE',  ( -0.000000000000000000, -0.000000000000000000, 1.000000000000000000 ) ) ;
#19936=DIRECTION ( 'NONE',  ( 0.9435911131814398445, -0.3311129884571295534, 0.000000000000000000 ) ) ;
#19940=EDGE_LOOP ( 'NONE', ( #26208, #4242, #3116, #6947 ) ) ;
#19969=EDGE_LOOP ( 'NONE', ( #1422, #8990, #34213, #24866 ) ) ;
#19986=ORIENTED_EDGE ( 'NONE', *, *, #13792, .F. ) ;
#19988=VECTOR ( 'NONE', #38224, 1000.000000000000000 ) ;
#20006=CARTESIAN_POINT ( 'NONE',  ( -15.44521549751111955, -137.7748507232956001, -2.500000000000000000 ) ) ;
#20019=DIRECTION ( 'NONE',  ( -0.000000000000000000, -0.000000000000000000, -1.000000000000000000 ) ) ;
#20042=SURFACE_SIDE_STYLE ('',( #1454 ) ) ;
#20051=ADVANCED_FACE ( 'NONE', ( #3456, #33323 ), #44821, .F. ) ;
#20073=PLANE ( 'NONE',  #9489 ) ;
#20079=ORIENTED_EDGE ( 'NONE', *, *, #27471, .F. ) ;
#20080=LINE ( 'NONE', #21035, #41472 ) ;
#20100=LINE ( 'NONE', #12523, #41239 ) ;
#20102=CARTESIAN_POINT ( 'NONE',  ( 18.80329974962065265, -105.8248132807389084, 5.500000000000000000 ) ) ;
#20114=VECTOR ( 'NONE', #2880, 1000.000000000000000 ) ;
#20139=ORIENTED_EDGE ( 'NONE', *, *, #12109, .T. ) ;
#20149=ORIENTED_EDGE ( 'NONE', *, *, #39352, .T. ) ;
#20153=LINE ( 'NONE', #5465, #31482 ) ;
#20156=DIRECTION ( 'NONE',  ( 0.9966891607226785466, 0.08130631524009969413, 0.000000000000000000 ) ) ;
#20158=CARTESIAN_POINT ( 'NONE',  ( -17.26469406256017791, -140.1601175325492648, -5.500000000000000000 ) ) ;
#20161=AXIS2_PLACEMENT_3D ( 'NONE', #38091, #19458, #45920 ) ;
#20167=LINE ( 'NONE', #2067, #44750 ) ;
#20173=EDGE_CURVE ( 'NONE', #28952, #12242, #46037, .T. ) ;
#20194=ORIENTED_EDGE ( 'NONE', *, *, #37446, .F. ) ;
#20196=DIRECTION ( 'NONE',  ( 0.000000000000000000, 0.000000000000000000, -1.000000000000000000 ) ) ;
#20210=EDGE_CURVE ( 'NONE', #10102, #20931, #39420, .T. ) ;
#20216=CARTESIAN_POINT ( 'NONE',  ( -7.572224309238338336, -145.4393675041377492, 2.500000000000000000 ) ) ;
#20233=ORIENTED_EDGE ( 'NONE', *, *, #41303, .T. ) ;
#20234=ORIENTED_EDGE ( 'NONE', *, *, #5938, .F. ) ;
#20235=DIRECTION ( 'NONE',  ( -0.000000000000000000, -0.000000000000000000, -1.000000000000000000 ) ) ;
#20250=EDGE_LOOP ( 'NONE', ( #21597, #5425, #15156, #21303 ) ) ;
#20259=VERTEX_POINT ( 'NONE', #43796 ) ;
#20275=DIRECTION ( 'NONE',  ( 0.9435911131814395114, -0.3311129884571304971, 0.000000000000000000 ) ) ;
#20319=DIRECTION ( 'NONE',  ( -1.000000000000000000, 0.000000000000000000, 0.000000000000000000 ) ) ;
#20320=ADVANCED_FACE ( 'NONE', ( #37421 ), #30087, .F. ) ;
#20351=ORIENTED_EDGE ( 'NONE', *, *, #18561, .T. ) ;
#20360=PLANE ( 'NONE',  #17327 ) ;
#20367=VECTOR ( 'NONE', #2361, 1000.000000000000114 ) ;
#20377=DIRECTION ( 'NONE',  ( 0.000000000000000000, 0.000000000000000000, 1.000000000000000000 ) ) ;
#20397=CARTESIAN_POINT ( 'NONE',  ( -23.97194136764370498, -131.3950000906648938, 5.500000000000000000 ) ) ;
#20400=ADVANCED_FACE ( 'NONE', ( #26651 ), #6840, .F. ) ;
#20425=ORIENTED_EDGE ( 'NONE', *, *, #44542, .F. ) ;
#20446=ADVANCED_FACE ( 'NONE', ( #27617 ), #12219, .F. ) ;
#20460=AXIS2_PLACEMENT_3D ( 'NONE', #42058, #16584, #35178 ) ;
#20465=VERTEX_POINT ( 'NONE', #45986 ) ;
#20468=DIRECTION ( 'NONE',  ( -0.02332147558787930897, -0.9997280174009348652, 0.000000000000000000 ) ) ;
#20477=EDGE_LOOP ( 'NONE', ( #21431, #9881, #7709, #43735 ) ) ;
#20496=EDGE_LOOP ( 'NONE', ( #25345, #46856, #29047, #36828 ) ) ;
#20504=EDGE_CURVE ( 'NONE', #35598, #17038, #46468, .T. ) ;
#20508=DIRECTION ( 'NONE',  ( -0.000000000000000000, -0.000000000000000000, 1.000000000000000000 ) ) ;
#20533=ORIENTED_EDGE ( 'NONE', *, *, #28958, .F. ) ;
#20537=VECTOR ( 'NONE', #23526, 1000.000000000000000 ) ;
#20548=ADVANCED_FACE ( 'NONE', ( #34222 ), #693, .F. ) ;
#20560=ORIENTED_EDGE ( 'NONE', *, *, #8962, .T. ) ;
#20577=DIRECTION ( 'NONE',  ( -0.000000000000000000, -0.000000000000000000, 1.000000000000000000 ) ) ;
#20585=DIRECTION ( 'NONE',  ( 0.6862798483830554463, 0.7273375899149793211, -0.000000000000000000 ) ) ;
#20611=EDGE_CURVE ( 'NONE', #33987, #46736, #25134, .T. ) ;
#20646=LINE ( 'NONE', #24807, #4294 ) ;
#20663=VECTOR ( 'NONE', #44057, 1000.000000000000114 ) ;
#20666=VECTOR ( 'NONE', #31807, 1000.000000000000000 ) ;
#20674=VECTOR ( 'NONE', #31008, 1000.000000000000227 ) ;
#20676=CARTESIAN_POINT ( 'NONE',  ( -0.9515373497862389396, -96.47140937769621871, 2.500000000000000000 ) ) ;
#20683=EDGE_CURVE ( 'NONE', #6225, #32049, #24901, .T. ) ;
#20690=CARTESIAN_POINT ( 'NONE',  ( 16.84844760790522145, -103.5491698323862124, -2.500000000000000000 ) ) ;
#20702=FACE_OUTER_BOUND ( 'NONE', #28507, .T. ) ;
#20706=AXIS2_PLACEMENT_3D ( 'NONE', #43904, #40485, #36556 ) ;
#20709=DIRECTION ( 'NONE',  ( 0.2867529058022035837, -0.9580045777625452175, 0.000000000000000000 ) ) ;
#20711=VECTOR ( 'NONE', #15826, 1000.000000000000114 ) ;
#20719=EDGE_LOOP ( 'NONE', ( #3371, #576, #16931, #22294 ) ) ;
#20728=ORIENTED_EDGE ( 'NONE', *, *, #28958, .T. ) ;
#20756=VERTEX_POINT ( 'NONE', #21945 ) ;
#20758=CARTESIAN_POINT ( 'NONE',  ( 16.30584220631899228, -140.9432449716519784, -5.500000000000000000 ) ) ;
#20765=VECTOR ( 'NONE', #39274, 1000.000000000000000 ) ;
#20769=ADVANCED_FACE ( 'NONE', ( #22675 ), #18991, .F. ) ;
#20792=EDGE_LOOP ( 'NONE', ( #8729, #27053, #15949, #7435 ) ) ;
#20801=LINE ( 'NONE', #32069, #30595 ) ;
#20837=ORIENTED_EDGE ( 'NONE', *, *, #28624, .F. ) ;
#20843=DIRECTION ( 'NONE',  ( -0.7273375899149793211, 0.6862798483830554463, 0.000000000000000000 ) ) ;
#20846=EDGE_CURVE ( 'NONE', #551, #20465, #14374, .T. ) ;
#20847=ORIENTED_EDGE ( 'NONE', *, *, #34926, .F. ) ;
#20850=VERTEX_POINT ( 'NONE', #22196 ) ;
#20859=DIRECTION ( 'NONE',  ( 0.8225049752423776450, 0.5687579148473765889, -0.000000000000000000 ) ) ;
#20861=EDGE_LOOP ( 'NONE', ( #38186, #44253, #10391, #22059 ) ) ;
#20896=DIRECTION ( 'NONE',  ( 0.000000000000000000, 0.000000000000000000, 1.000000000000000000 ) ) ;
#20898=EDGE_CURVE ( 'NONE', #34042, #11749, #11669, .T. ) ;
#20931=VERTEX_POINT ( 'NONE', #45929 ) ;
#20933=CARTESIAN_POINT ( 'NONE',  ( 6.377742925735834234, -145.7647898336707897, -2.500000000000000000 ) ) ;
#20949=CIRCLE ( 'NONE', #6108, 35.50000000000000711 ) ;
#20958=ORIENTED_EDGE ( 'NONE', *, *, #19805, .F. ) ;
#20965=VECTOR ( 'NONE', #30108, 1000.000000000000000 ) ;
#20966=ORIENTED_EDGE ( 'NONE', *, *, #17344, .F. ) ;
#20978=DIRECTION ( 'NONE',  ( 0.3090169943749573878, -0.9510565162951503115, 0.000000000000000000 ) ) ;
#20986=LINE ( 'NONE', #17790, #29924 ) ;
#20989=ORIENTED_EDGE ( 'NONE', *, *, #46447, .F. ) ;
#21000=CARTESIAN_POINT ( 'NONE',  ( -25.50183398199384754, -112.6408924756582053, 5.500000000000000000 ) ) ;
#21003=DIRECTION ( 'NONE',  ( -0.000000000000000000, -0.000000000000000000, -1.000000000000000000 ) ) ;
#21013=CARTESIAN_POINT ( 'NONE',  ( -23.30023580412278505, -123.4057321492263384, -5.500000000000000000 ) ) ;
#21019=VECTOR ( 'NONE', #36162, 1000.000000000000000 ) ;
#21021=VERTEX_POINT ( 'NONE', #28274 ) ;
#21032=ORIENTED_EDGE ( 'NONE', *, *, #3501, .T. ) ;
#21034=VERTEX_POINT ( 'NONE', #43465 ) ;
#21035=CARTESIAN_POINT ( 'NONE',  ( -20.30386590532152979, -102.9045904027214959, -5.500000000000000000 ) ) ;
#21038=ORIENTED_EDGE ( 'NONE', *, *, #28624, .T. ) ;
#21048=EDGE_CURVE ( 'NONE', #33987, #25896, #43689, .T. ) ;
#21060=CARTESIAN_POINT ( 'NONE',  ( -21.33958957442910886, -129.9559990355020034, -2.500000000000000000 ) ) ;
#21061=VERTEX_POINT ( 'NONE', #28529 ) ;
#21063=DIRECTION ( 'NONE',  ( -0.000000000000000000, -0.000000000000000000, 1.000000000000000000 ) ) ;
#21064=ADVANCED_FACE ( 'NONE', ( #24614 ), #21166, .F. ) ;
#21080=EDGE_CURVE ( 'NONE', #41947, #37711, #35859, .T. ) ;
#21106=AXIS2_PLACEMENT_3D ( 'NONE', #8923, #23860, #42949 ) ;
#21109=CARTESIAN_POINT ( 'NONE',  ( 21.07894319797337701, -103.8699611390234878, 5.500000000000000000 ) ) ;
#21124=EDGE_CURVE ( 'NONE', #24556, #17554, #35629, .T. ) ;
#21129=ORIENTED_EDGE ( 'NONE', *, *, #11621, .T. ) ;
#21141=FACE_OUTER_BOUND ( 'NONE', #13258, .T. ) ;
#21147=DIRECTION ( 'NONE',  ( -0.9997280174009349762, 0.02332147558787671729, 0.000000000000000000 ) ) ;
#21153=EDGE_LOOP ( 'NONE', ( #18470, #23859, #21998, #21590 ) ) ;
#21166=PLANE ( 'NONE',  #45500 ) ;
#21178=ORIENTED_EDGE ( 'NONE', *, *, #7578, .F. ) ;
#21201=VECTOR ( 'NONE', #29660, 1000.000000000000114 ) ;
#21211=FACE_BOUND ( 'NONE', #36963, .T. ) ;
#21213=DIRECTION ( 'NONE',  ( -0.000000000000000000, -0.000000000000000000, -1.000000000000000000 ) ) ;
#21232=ADVANCED_FACE ( 'NONE', ( #14313 ), #40274, .F. ) ;
#21233=LINE ( 'NONE', #10224, #25531 ) ;
#21240=VECTOR ( 'NONE', #44716, 1000.000000000000000 ) ;
#21248=EDGE_CURVE ( 'NONE', #4261, #20756, #21658, .T. ) ;
#21251=EDGE_CURVE ( 'NONE', #24549, #43507, #36582, .T. ) ;
#21260=EDGE_CURVE ( 'NONE', #28358, #35358, #36815, .T. ) ;
#21261=VERTEX_POINT ( 'NONE', #11126 ) ;
#21266=ORIENTED_EDGE ( 'NONE', *, *, #19536, .F. ) ;
#21281=DIRECTION ( 'NONE',  ( 0.8774505977381971134, 0.4796670183876317051, -0.000000000000000000 ) ) ;
#21292=CARTESIAN_POINT ( 'NONE',  ( 19.29194287201271862, -133.5026271600380880, 5.500000000000000000 ) ) ;
#21295=LINE ( 'NONE', #3668, #42041 ) ;
#21303=ORIENTED_EDGE ( 'NONE', *, *, #38695, .T. ) ;
#21305=EDGE_CURVE ( 'NONE', #28952, #38166, #36930, .T. ) ;
#21313=EDGE_LOOP ( 'NONE', ( #47974, #43117, #12509, #30870 ) ) ;
#21321=DIRECTION ( 'NONE',  ( 0.4796670183876317051, -0.8774505977381972244, 0.000000000000000000 ) ) ;
#21334=VERTEX_POINT ( 'NONE', #27031 ) ;
#21358=CARTESIAN_POINT ( 'NONE',  ( -13.05994868825747446, -139.5943292883446532, 5.500000000000000000 ) ) ;
#21376=ADVANCED_FACE ( 'NONE', ( #37790 ), #41964, .F. ) ;
#21377=DIRECTION ( 'NONE',  ( -0.8090169943749504489, 0.5877852522924689183, 0.000000000000000000 ) ) ;
#21379=EDGE_CURVE ( 'NONE', #12299, #25561, #19187, .T. ) ;
#21383=CARTESIAN_POINT ( 'NONE',  ( 5.822613034544236399, -142.8165987265839760, -5.500000000000000000 ) ) ;
#21395=CARTESIAN_POINT ( 'NONE',  ( 23.41451323550360186, -132.5004227906269989, 5.500000000000000000 ) ) ;
#21406=LINE ( 'NONE', #9193, #38536 ) ;
#21415=CARTESIAN_POINT ( 'NONE',  ( 16.84844760790522855, -103.5491698323862124, -5.500000000000000000 ) ) ;
#21431=ORIENTED_EDGE ( 'NONE', *, *, #35086, .F. ) ;
#21452=ORIENTED_EDGE ( 'NONE', *, *, #30261, .T. ) ;
#21463=VECTOR ( 'NONE', #31731, 1000.000000000000114 ) ;
#21470=FILL_AREA_STYLE_COLOUR ( '', #12500 ) ;
#21477=ORIENTED_EDGE ( 'NONE', *, *, #28636, .F. ) ;
#21479=AXIS2_PLACEMENT_3D ( 'NONE', #14736, #37242, #11313 ) ;
#21495=EDGE_CURVE ( 'NONE', #4190, #42528, #20153, .T. ) ;
#21517=CARTESIAN_POINT ( 'NONE',  ( 2.874421927457452952, -143.3717286177755739, 5.500000000000000000 ) ) ;
#21538=PLANE ( 'NONE',  #75 ) ;
#21561=VECTOR ( 'NONE', #33167, 1000.000000000000114 ) ;
#21585=LINE ( 'NONE', #14234, #26282 ) ;
#21590=ORIENTED_EDGE ( 'NONE', *, *, #24155, .F. ) ;
#21597=ORIENTED_EDGE ( 'NONE', *, *, #42796, .F. ) ;
#21606=DIRECTION ( 'NONE',  ( -0.02332147558787823691, -0.9997280174009349762, 0.000000000000000000 ) ) ;
#21619=EDGE_CURVE ( 'NONE', #8377, #36404, #29367, .T. ) ;
#21620=ORIENTED_EDGE ( 'NONE', *, *, #47504, .T. ) ;
#21634=PLANE ( 'NONE',  #37025 ) ;
#21639=VERTEX_POINT ( 'NONE', #30097 ) ;
#21642=DIRECTION ( 'NONE',  ( -1.000000000000000000, 0.000000000000000000, 0.000000000000000000 ) ) ;
#21646=DIRECTION ( 'NONE',  ( 0.8541291221503261033, -0.5200609990133016058, 0.000000000000000000 ) ) ;
#21658=LINE ( 'NONE', #14799, #13472 ) ;
#21665=DIRECTION ( 'NONE',  ( -0.7273375899149812085, 0.6862798483830533369, 0.000000000000000000 ) ) ;
#21668=CARTESIAN_POINT ( 'NONE',  ( -0.8815729230226008184, -93.47222532549339746, 5.500000000000000000 ) ) ;
#21676=CARTESIAN_POINT ( 'NONE',  ( 13.83832728059186046, -142.6495187161941089, 5.500000000000000000 ) ) ;
#21684=ORIENTED_EDGE ( 'NONE', *, *, #15873, .F. ) ;
#21693=ORIENTED_EDGE ( 'NONE', *, *, #13169, .F. ) ;
#21706=FACE_BOUND ( 'NONE', #14315, .T. ) ;
#21715=LINE ( 'NONE', #36638, #17101 ) ;
#21725=CARTESIAN_POINT ( 'NONE',  ( 0.000000000000000000, -120.0000000000000000, 2.500000000000000000 ) ) ;
#21732=ORIENTED_EDGE ( 'NONE', *, *, #30655, .T. ) ;
#21739=DIRECTION ( 'NONE',  ( 0.000000000000000000, 0.000000000000000000, 1.000000000000000000 ) ) ;
#21747=EDGE_LOOP ( 'NONE', ( #11429, #31544, #34212, #36276 ) ) ;
#21754=VERTEX_POINT ( 'NONE', #8767 ) ;
#21756=VECTOR ( 'NONE', #26986, 1000.000000000000000 ) ;
#21760=EDGE_LOOP ( 'NONE', ( #42993, #7309, #31592, #34603 ) ) ;
#21761=PLANE ( 'NONE',  #25205 ) ;
#21785=ORIENTED_EDGE ( 'NONE', *, *, #2808, .T. ) ;
#21789=ORIENTED_EDGE ( 'NONE', *, *, #4651, .F. ) ;
#21809=VERTEX_POINT ( 'NONE', #39125 ) ;
#21817=EDGE_LOOP ( 'NONE', ( #31909, #48364, #12153, #14606 ) ) ;
#21822=DIRECTION ( 'NONE',  ( -0.000000000000000000, -0.000000000000000000, -1.000000000000000000 ) ) ;
#21826=CARTESIAN_POINT ( 'NONE',  ( -6.880223345695647197, -142.5202692415819854, 5.500000000000000000 ) ) ;
#21835=CARTESIAN_POINT ( 'NONE',  ( 19.12409105625795291, -101.5943176906707919, 2.500000000000000000 ) ) ;
#21838=CARTESIAN_POINT ( 'NONE',  ( -0.4301293587032979371, -118.5629931333561871, -2.500000000000000000 ) ) ;
#21853=ORIENTED_EDGE ( 'NONE', *, *, #8780, .T. ) ;
#21858=FACE_OUTER_BOUND ( 'NONE', #42337, .T. ) ;
#21860=VERTEX_POINT ( 'NONE', #24909 ) ;
#21869=VECTOR ( 'NONE', #26179, 1000.000000000000114 ) ;
#21886=CARTESIAN_POINT ( 'NONE',  ( 14.59956846177685996, -138.4757300459248484, -5.500000000000000000 ) ) ;
#21912=ORIENTED_EDGE ( 'NONE', *, *, #46447, .T. ) ;
#21936=CARTESIAN_POINT ( 'NONE',  ( 24.95699195200416654, -110.9640411295978595, -5.500000000000000000 ) ) ;
#21939=FACE_BOUND ( 'NONE', #40366, .T. ) ;
#21941=DIRECTION ( 'NONE',  ( -0.000000000000000000, -0.000000000000000000, -1.000000000000000000 ) ) ;
#21943=CARTESIAN_POINT ( 'NONE',  ( 3.429551818649054340, -146.3199197248623875, -5.500000000000000000 ) ) ;
#21945=CARTESIAN_POINT ( 'NONE',  ( 18.80329974962065265, -105.8248132807389084, 2.500000000000000000 ) ) ;
#21959=CARTESIAN_POINT ( 'NONE',  ( -18.12185313557660038, -104.9634299478706794, 5.500000000000000000 ) ) ;
#21980=ADVANCED_FACE ( 'NONE', ( #13901 ), #11676, .F. ) ;
#21985=DIRECTION ( 'NONE',  ( -0.000000000000000000, -0.000000000000000000, 1.000000000000000000 ) ) ;
#21990=ORIENTED_EDGE ( 'NONE', *, *, #11593, .F. ) ;
#21992=CARTESIAN_POINT ( 'NONE',  ( -22.67106064244953245, -113.6342314410295842, 5.500000000000000000 ) ) ;
#21995=ORIENTED_EDGE ( 'NONE', *, *, #24897, .T. ) ;
#21998=ORIENTED_EDGE ( 'NONE', *, *, #38925, .F. ) ;
#21999=VERTEX_POINT ( 'NONE', #33223 ) ;
#22005=LINE ( 'NONE', #33022, #7029 ) ;
#22008=AXIS2_PLACEMENT_3D ( 'NONE', #32970, #44242, #29548 ) ;
#22021=EDGE_CURVE ( 'NONE', #15663, #28440, #11452, .T. ) ;
#22030=DIRECTION ( 'NONE',  ( -0.000000000000000000, -0.000000000000000000, -1.000000000000000000 ) ) ;
#22035=DIRECTION ( 'NONE',  ( 0.6064928550163531940, 0.7950889364178782559, 0.000000000000000000 ) ) ;
#22059=ORIENTED_EDGE ( 'NONE', *, *, #8358, .T. ) ;
#22061=CARTESIAN_POINT ( 'NONE',  ( -13.05994868825747446, -139.5943292883446532, -2.500000000000000000 ) ) ;
#22067=PLANE ( 'NONE',  #35263 ) ;
#22106=CARTESIAN_POINT ( 'NONE',  ( 35.50000000000000711, -120.0000000000000000, 2.500000000000000000 ) ) ;
#22128=CARTESIAN_POINT ( 'NONE',  ( -21.33958957442910886, -129.9559990355020034, 2.500000000000000000 ) ) ;
#22145=DIRECTION ( 'NONE',  ( -0.6516173805718079581, 0.7585478161175704948, 0.000000000000000000 ) ) ;
#22146=CARTESIAN_POINT ( 'NONE',  ( -6.880223345695647197, -142.5202692415819854, 5.500000000000000000 ) ) ;
#22151=EDGE_CURVE ( 'NONE', #20259, #28619, #31494, .T. ) ;
#22152=VERTEX_POINT ( 'NONE', #20216 ) ;
#22170=FACE_OUTER_BOUND ( 'NONE', #19969, .T. ) ;
#22175=ORIENTED_EDGE ( 'NONE', *, *, #27187, .F. ) ;
#22190=CARTESIAN_POINT ( 'NONE',  ( -22.67106064244953245, -113.6342314410295842, 2.500000000000000000 ) ) ;
#22196=CARTESIAN_POINT ( 'NONE',  ( 23.41451323550360186, -132.5004227906269989, -5.500000000000000000 ) ) ;
#22218=CARTESIAN_POINT ( 'NONE',  ( 6.377742925735834234, -145.7647898336708181, 5.500000000000000000 ) ) ;
#22231=ORIENTED_EDGE ( 'NONE', *, *, #35301, .F. ) ;
#22261=FACE_OUTER_BOUND ( 'NONE', #24878, .T. ) ;
#22262=DIRECTION ( 'NONE',  ( -0.08130631524010117905, 0.9966891607226784355, 0.000000000000000000 ) ) ;
#22268=ADVANCED_FACE ( 'NONE', ( #8240 ), #38108, .F. ) ;
#22279=ORIENTED_EDGE ( 'NONE', *, *, #21124, .T. ) ;
#22280=VECTOR ( 'NONE', #29461, 1000.000000000000000 ) ;
#22294=ORIENTED_EDGE ( 'NONE', *, *, #18947, .T. ) ;
#22303=EDGE_LOOP ( 'NONE', ( #32046, #14049, #41442, #13446 ) ) ;
#22307=ORIENTED_EDGE ( 'NONE', *, *, #9230, .F. ) ;
#22312=CARTESIAN_POINT ( 'NONE',  ( -18.24502636017238899, -100.7225776329765665, 5.500000000000000000 ) ) ;
#22315=ADVANCED_FACE ( 'NONE', ( #24852 ), #17252, .F. ) ;
#22319=DIRECTION ( 'NONE',  ( 0.8225049752423776450, 0.5687579148473764779, 0.000000000000000000 ) ) ;
#22322=CARTESIAN_POINT ( 'NONE',  ( 16.30584220631899228, -140.9432449716519784, 5.500000000000000000 ) ) ;
#22337=CARTESIAN_POINT ( 'NONE',  ( -0.9515373497862389396, -96.47140937769621871, 5.500000000000000000 ) ) ;
#22347=VECTOR ( 'NONE', #4461, 1000.000000000000000 ) ;
#22358=ORIENTED_EDGE ( 'NONE', *, *, #25861, .F. ) ;
#22361=FACE_OUTER_BOUND ( 'NONE', #45756, .T. ) ;
#22369=DIRECTION ( 'NONE',  ( -0.000000000000000000, -0.000000000000000000, -1.000000000000000000 ) ) ;
#22373=EDGE_CURVE ( 'NONE', #25110, #21860, #2333, .T. ) ;
#22382=CARTESIAN_POINT ( 'NONE',  ( 23.41451323550360186, -132.5004227906269989, 5.500000000000000000 ) ) ;
#22409=EDGE_CURVE ( 'NONE', #28111, #39825, #31748, .T. ) ;
#22441=LINE ( 'NONE', #44463, #25256 ) ;
#22448=ORIENTED_EDGE ( 'NONE', *, *, #1148, .F. ) ;
#22467=FACE_OUTER_BOUND ( 'NONE', #35875, .T. ) ;
#22480=VERTEX_POINT ( 'NONE', #33407 ) ;
#22517=LINE ( 'NONE', #23240, #38939 ) ;
#22558=ORIENTED_EDGE ( 'NONE', *, *, #9995, .F. ) ;
#22568=DIRECTION ( 'NONE',  ( -0.5687579148473765889, 0.8225049752423776450, 0.000000000000000000 ) ) ;
#22573=LINE ( 'NONE', #21838, #296 ) ;
#22575=CARTESIAN_POINT ( 'NONE',  ( -23.30023580412278505, -123.4057321492263384, 5.500000000000000000 ) ) ;
#22578=ORIENTED_EDGE ( 'NONE', *, *, #36080, .F. ) ;
#22589=ADVANCED_FACE ( 'NONE', ( #4751 ), #4995, .F. ) ;
#22592=DIRECTION ( 'NONE',  ( -0.000000000000000000, -0.000000000000000000, -1.000000000000000000 ) ) ;
#22597=EDGE_CURVE ( 'NONE', #10969, #23846, #8648, .T. ) ;
#22600=CARTESIAN_POINT ( 'NONE',  ( -23.54415474984308432, -120.4156646670583086, -2.500000000000000000 ) ) ;
#22607=ORIENTED_EDGE ( 'NONE', *, *, #15798, .F. ) ;
#22611=DIRECTION ( 'NONE',  ( -0.6862798483830544471, -0.7273375899149802093, 0.000000000000000000 ) ) ;
#22638=ORIENTED_EDGE ( 'NONE', *, *, #23652, .T. ) ;
#22661=VECTOR ( 'NONE', #18389, 1000.000000000000000 ) ;
#22663=VERTEX_POINT ( 'NONE', #46117 ) ;
#22675=FACE_OUTER_BOUND ( 'NONE', #35145, .T. ) ;
#22696=AXIS2_PLACEMENT_3D ( 'NONE', #33788, #22784, #34761 ) ;
#22711=CARTESIAN_POINT ( 'NONE',  ( -23.54415474984308787, -120.4156646670583086, 5.500000000000000000 ) ) ;
#22730=VECTOR ( 'NONE', #44467, 1000.000000000000000 ) ;
#22731=EDGE_LOOP ( 'NONE', ( #149, #21995, #47353, #41332 ) ) ;
#22735=FACE_OUTER_BOUND ( 'NONE', #37963, .T. ) ;
#22742=DIRECTION ( 'NONE',  ( 0.7585478161175723821, 0.6516173805718057377, 0.000000000000000000 ) ) ;
#22745=CARTESIAN_POINT ( 'NONE',  ( -17.26469406256017791, -140.1601175325492648, 2.500000000000000000 ) ) ;
#22746=CARTESIAN_POINT ( 'NONE',  ( 18.80329974962065265, -105.8248132807389084, -2.500000000000000000 ) ) ;
#22759=AXIS2_PLACEMENT_3D ( 'NONE', #16361, #31547, #19516 ) ;
#22766=ORIENTED_EDGE ( 'NONE', *, *, #46913, .F. ) ;
#22768=EDGE_LOOP ( 'NONE', ( #513, #14229, #43455, #21732 ) ) ;
#22784=DIRECTION ( 'NONE',  ( 1.000000000000000000, 0.000000000000000000, -0.000000000000000000 ) ) ;
#22794=ORIENTED_EDGE ( 'NONE', *, *, #28735, .F. ) ;
#22803=EDGE_CURVE ( 'NONE', #37711, #15663, #39249, .T. ) ;
#22811=LINE ( 'NONE', #7156, #2542 ) ;
#22819=ORIENTED_EDGE ( 'NONE', *, *, #9889, .F. ) ;
#22828=EDGE_CURVE ( 'NONE', #18661, #29809, #22573, .T. ) ;
#22879=AXIS2_PLACEMENT_3D ( 'NONE', #25914, #40142, #43800 ) ;
#22888=CARTESIAN_POINT ( 'NONE',  ( 23.11608002360578240, -124.4885236261218182, -2.500000000000000000 ) ) ;
#22892=ORIENTED_EDGE ( 'NONE', *, *, #41620, .F. ) ;
#22901=ORIENTED_EDGE ( 'NONE', *, *, #21379, .F. ) ;
#22948=ORIENTED_EDGE ( 'NONE', *, *, #2641, .T. ) ;
#22950=ORIENTED_EDGE ( 'NONE', *, *, #45166, .F. ) ;
#22955=CARTESIAN_POINT ( 'NONE',  ( 9.984461079971730157, -95.40710393340120277, 2.500000000000000000 ) ) ;
#22975=LINE ( 'NONE', #4140, #4863 ) ;
#22993=( LENGTH_UNIT ( ) NAMED_UNIT ( * ) SI_UNIT ( .MILLI., .METRE. ) );
#22997=ORIENTED_EDGE ( 'NONE', *, *, #5938, .T. ) ;
#22998=VECTOR ( 'NONE', #48201, 1000.000000000000000 ) ;
#23014=ORIENTED_EDGE ( 'NONE', *, *, #12001, .F. ) ;
#23019=ORIENTED_EDGE ( 'NONE', *, *, #38911, .F. ) ;
#23040=CARTESIAN_POINT ( 'NONE',  ( 21.85433023846371370, -135.0628101570779620, -5.500000000000000000 ) ) ;
#23048=AXIS2_PLACEMENT_3D ( 'NONE', #4159, #27836, #44780 ) ;
#23052=FACE_OUTER_BOUND ( 'NONE', #29675, .T. ) ;
#23075=VECTOR ( 'NONE', #4540, 999.9999999999998863 ) ;
#23093=EDGE_LOOP ( 'NONE', ( #25310, #12968, #35418, #8757 ) ) ;
#23103=PLANE ( 'NONE',  #29987 ) ;
#23118=CARTESIAN_POINT ( 'NONE',  ( -25.50183398199384754, -112.6408924756582053, 5.500000000000000000 ) ) ;
#23131=AXIS2_PLACEMENT_3D ( 'NONE', #4962, #46090, #4720 ) ;
#23133=VECTOR ( 'NONE', #45550, 1000.000000000000000 ) ;
#23136=CARTESIAN_POINT ( 'NONE',  ( -23.54415474984308787, -120.4156646670583086, 5.500000000000000000 ) ) ;
#23142=ORIENTED_EDGE ( 'NONE', *, *, #18913, .F. ) ;
#23160=VERTEX_POINT ( 'NONE', #9095 ) ;
#23170=CARTESIAN_POINT ( 'NONE',  ( -7.670864526094549163, -97.73662565058241114, 5.500000000000000000 ) ) ;
#23178=AXIS2_PLACEMENT_3D ( 'NONE', #42081, #38403, #44776 ) ;
#23180=LINE ( 'NONE', #12648, #2919 ) ;
#23185=ORIENTED_EDGE ( 'NONE', *, *, #47665, .T. ) ;
#23188=DIRECTION ( 'NONE',  ( -0.4279312458752990711, -0.9038112904824846527, 0.000000000000000000 ) ) ;
#23203=EDGE_LOOP ( 'NONE', ( #38907, #12867, #44394, #21038 ) ) ;
#23237=DIRECTION ( 'NONE',  ( -0.000000000000000000, -0.000000000000000000, -1.000000000000000000 ) ) ;
#23240=CARTESIAN_POINT ( 'NONE',  ( -3.961125083139900749, -143.2122702051246677, 5.500000000000000000 ) ) ;
#23241=ORIENTED_EDGE ( 'NONE', *, *, #30792, .T. ) ;
#23254=EDGE_LOOP ( 'NONE', ( #3000, #449, #44288, #24151 ) ) ;
#23256=VECTOR ( 'NONE', #28826, 1000.000000000000114 ) ;
#23257=ORIENTED_EDGE ( 'NONE', *, *, #26413, .F. ) ;
#23258=EDGE_LOOP ( 'NONE', ( #10788, #45326, #1667, #31109 ) ) ;
#23267=ORIENTED_EDGE ( 'NONE', *, *, #33378, .F. ) ;
#23268=CARTESIAN_POINT ( 'NONE',  ( 8.700667342345820288, -98.11853780484867116, 5.500000000000000000 ) ) ;
#23283=DIRECTION ( 'NONE',  ( -0.000000000000000000, -0.000000000000000000, 1.000000000000000000 ) ) ;
#23287=DIRECTION ( 'NONE',  ( -0.000000000000000000, -0.000000000000000000, -1.000000000000000000 ) ) ;
#23307=ORIENTED_EDGE ( 'NONE', *, *, #42609, .F. ) ;
#23313=EDGE_LOOP ( 'NONE', ( #10073, #37101, #32433, #39894 ) ) ;
#23317=LINE ( 'NONE', #4487, #27820 ) ;
#23324=EDGE_CURVE ( 'NONE', #18975, #11732, #39914, .T. ) ;
#23330=EDGE_LOOP ( 'NONE', ( #43393, #12617, #42226, #392 ) ) ;
#23331=EDGE_CURVE ( 'NONE', #16986, #26232, #29120, .T. ) ;
#23334=LINE ( 'NONE', #16479, #6322 ) ;
#23336=ORIENTED_EDGE ( 'NONE', *, *, #31011, .F. ) ;
#23337=DIRECTION ( 'NONE',  ( -0.000000000000000000, -0.000000000000000000, -1.000000000000000000 ) ) ;
#23350=EDGE_LOOP ( 'NONE', ( #31163, #21178, #27972, #26497 ) ) ;
#23360=EDGE_CURVE ( 'NONE', #45107, #34199, #10283, .T. ) ;
#23395=DIRECTION ( 'NONE',  ( -0.000000000000000000, -0.000000000000000000, -1.000000000000000000 ) ) ;
#23399=CARTESIAN_POINT ( 'NONE',  ( -3.961125083139900749, -143.2122702051246677, 5.500000000000000000 ) ) ;
#23400=CARTESIAN_POINT ( 'NONE',  ( -9.055038557894883766, -98.31460683512894150, 2.500000000000000000 ) ) ;
#23414=EDGE_LOOP ( 'NONE', ( #40694, #5444, #7071, #40046 ) ) ;
#23423=VERTEX_POINT ( 'NONE', #22745 ) ;
#23426=EDGE_CURVE ( 'NONE', #17612, #4369, #19312, .T. ) ;
#23428=LINE ( 'NONE', #13875, #26896 ) ;
#23463=ORIENTED_EDGE ( 'NONE', *, *, #45513, .T. ) ;
#23464=ADVANCED_FACE ( 'NONE', ( #15421 ), #34239, .F. ) ;
#23473=EDGE_CURVE ( 'NONE', #21639, #11732, #44145, .T. ) ;
#23480=EDGE_CURVE ( 'NONE', #41940, #34545, #26187, .T. ) ;
#23487=EDGE_LOOP ( 'NONE', ( #31355, #23463, #22638, #29248 ) ) ;
#23498=ORIENTED_EDGE ( 'NONE', *, *, #41792, .F. ) ;
#23512=FACE_OUTER_BOUND ( 'NONE', #37996, .T. ) ;
#23520=CARTESIAN_POINT ( 'NONE',  ( -26.29030328629082902, -123.6496510949466341, -2.500000000000000000 ) ) ;
#23524=VECTOR ( 'NONE', #42105, 1000.000000000000000 ) ;
#23526=DIRECTION ( 'NONE',  ( -0.000000000000000000, -0.000000000000000000, -1.000000000000000000 ) ) ;
#23531=ORIENTED_EDGE ( 'NONE', *, *, #9176, .F. ) ;
#23560=CARTESIAN_POINT ( 'NONE',  ( 20.85212586905261745, -130.9402397935870965, -2.500000000000000000 ) ) ;
#23577=DIRECTION ( 'NONE',  ( 0.9435911131814398445, -0.3311129884571295534, 0.000000000000000000 ) ) ;
#23580=CARTESIAN_POINT ( 'NONE',  ( -23.54415474984308787, -120.4156646670583086, 5.500000000000000000 ) ) ;
#23608=DIRECTION ( 'NONE',  ( 0.3853207896976547087, -0.9227826878668540234, 0.000000000000000000 ) ) ;
#23610=CARTESIAN_POINT ( 'NONE',  ( -15.44521549751111422, -137.7748507232956001, -5.500000000000000000 ) ) ;
#23622=ORIENTED_EDGE ( 'NONE', *, *, #5477, .F. ) ;
#23625=DIRECTION ( 'NONE',  ( -0.1850432970638667129, 0.9827303690289281857, 0.000000000000000000 ) ) ;
#23634=DIRECTION ( 'NONE',  ( -0.000000000000000000, -0.000000000000000000, -1.000000000000000000 ) ) ;
#23648=ADVANCED_FACE ( 'NONE', ( #14083 ), #10411, .T. ) ;
#23652=EDGE_CURVE ( 'NONE', #42694, #551, #24629, .T. ) ;
#23657=EDGE_CURVE ( 'NONE', #19570, #25110, #11397, .T. ) ;
#23661=ORIENTED_EDGE ( 'NONE', *, *, #47124, .F. ) ;
#23666=CARTESIAN_POINT ( 'NONE',  ( 22.94323693612312809, -114.6983135802921083, 2.500000000000000000 ) ) ;
#23700=LINE ( 'NONE', #34958, #12913 ) ;
#23715=CARTESIAN_POINT ( 'NONE',  ( -21.67772167707813935, -110.8034581014852762, 5.500000000000000000 ) ) ;
#23723=VECTOR ( 'NONE', #23237, 1000.000000000000000 ) ;
#23752=EDGE_LOOP ( 'NONE', ( #7496, #19337, #1656, #20149 ) ) ;
#23755=LINE ( 'NONE', #35013, #10380 ) ;
#23759=DIRECTION ( 'NONE',  ( 0.7950889364178796992, -0.6064928550163511956, 0.000000000000000000 ) ) ;
#23762=DIRECTION ( 'NONE',  ( -0.000000000000000000, -0.000000000000000000, -1.000000000000000000 ) ) ;
#23766=CARTESIAN_POINT ( 'NONE',  ( 16.84844760790522855, -103.5491698323862124, 5.500000000000000000 ) ) ;
#23767=DIRECTION ( 'NONE',  ( 0.8774505977381978905, 0.4796670183876304283, -0.000000000000000000 ) ) ;
#23769=EDGE_CURVE ( 'NONE', #26989, #18327, #29259, .T. ) ;
#23770=VECTOR ( 'NONE', #38271, 1000.000000000000114 ) ;
#23773=ADVANCED_FACE ( 'NONE', ( #110 ), #25573, .T. ) ;
#23801=ORIENTED_EDGE ( 'NONE', *, *, #5428, .F. ) ;
#23807=CARTESIAN_POINT ( 'NONE',  ( -13.05994868825747446, -139.5943292883446532, -5.500000000000000000 ) ) ;
#23827=ORIENTED_EDGE ( 'NONE', *, *, #17606, .T. ) ;
#23829=EDGE_CURVE ( 'NONE', #46921, #14358, #10576, .T. ) ;
#23836=DIRECTION ( 'NONE',  ( -0.000000000000000000, -0.000000000000000000, 1.000000000000000000 ) ) ;
#23839=DIRECTION ( 'NONE',  ( 0.9918136447140100120, -0.1276937514489704939, 0.000000000000000000 ) ) ;
#23843=ORIENTED_EDGE ( 'NONE', *, *, #12554, .T. ) ;
#23846=VERTEX_POINT ( 'NONE', #6181 ) ;
#23851=VECTOR ( 'NONE', #33414, 1000.000000000000000 ) ;
#23858=DIRECTION ( 'NONE',  ( 0.9997280174009349762, -0.02332147558787674158, 0.000000000000000000 ) ) ;
#23859=ORIENTED_EDGE ( 'NONE', *, *, #19482, .F. ) ;
#23860=DIRECTION ( 'NONE',  ( -0.08130631524009862554, 0.9966891607226787686, 0.000000000000000000 ) ) ;
#23903=VERTEX_POINT ( 'NONE', #2490 ) ;
#23907=VERTEX_POINT ( 'NONE', #35792 ) ;
#23916=ORIENTED_EDGE ( 'NONE', *, *, #34576, .T. ) ;
#23920=VECTOR ( 'NONE', #37289, 1000.000000000000114 ) ;
#23943=ORIENTED_EDGE ( 'NONE', *, *, #3796, .F. ) ;
#23969=DIRECTION ( 'NONE',  ( -0.9580045777625452175, -0.2867529058022035837, 0.000000000000000000 ) ) ;
#24009=ORIENTED_EDGE ( 'NONE', *, *, #26943, .F. ) ;
#24022=EDGE_LOOP ( 'NONE', ( #15082, #45781, #40357, #10443 ) ) ;
#24023=CARTESIAN_POINT ( 'NONE',  ( 32.50000000000000000, -120.0000000000000000, 2.500000000000000000 ) ) ;
#24036=DIRECTION ( 'NONE',  ( 0.000000000000000000, -1.000000000000000000, 0.000000000000000000 ) ) ;
#24061=CARTESIAN_POINT ( 'NONE',  ( -23.30023580412278861, -123.4057321492263384, -2.500000000000000000 ) ) ;
#24098=VECTOR ( 'NONE', #24397, 1000.000000000000114 ) ;
#24114=LINE ( 'NONE', #35113, #39184 ) ;
#24127=DIRECTION ( 'NONE',  ( 0.9997280174009349762, -0.02332147558787671729, 0.000000000000000000 ) ) ;
#24128=ORIENTED_EDGE ( 'NONE', *, *, #40242, .T. ) ;
#24132=DIRECTION ( 'NONE',  ( 0.4796670183876317051, -0.8774505977381971134, 0.000000000000000000 ) ) ;
#24151=ORIENTED_EDGE ( 'NONE', *, *, #36433, .T. ) ;
#24155=EDGE_CURVE ( 'NONE', #14947, #41627, #38929, .T. ) ;
#24161=AXIS2_PLACEMENT_3D ( 'NONE', #34426, #7544, #44985 ) ;
#24166=CARTESIAN_POINT ( 'NONE',  ( -23.54415474984308787, -120.4156646670583086, 5.500000000000000000 ) ) ;
#24208=DIRECTION ( 'NONE',  ( -0.3853207896976523772, 0.9227826878668550226, 0.000000000000000000 ) ) ;
#24248=LINE ( 'NONE', #8830, #44373 ) ;
#24253=LINE ( 'NONE', #9554, #36595 ) ;
#24269=VERTEX_POINT ( 'NONE', #31839 ) ;
#24274=CARTESIAN_POINT ( 'NONE',  ( 19.12409105625795291, -101.5943176906707919, 5.500000000000000000 ) ) ;
#24280=EDGE_LOOP ( 'NONE', ( #10620, #7610 ) ) ;
#24295=VERTEX_POINT ( 'NONE', #9523 ) ;
#24328=AXIS2_PLACEMENT_3D ( 'NONE', #12202, #15858, #27360 ) ;
#24330=ORIENTED_EDGE ( 'NONE', *, *, #21248, .T. ) ;
#24342=DIRECTION ( 'NONE',  ( 0.2306669878475637314, 0.9730327541852493711, -0.000000000000000000 ) ) ;
#24343=LINE ( 'NONE', #1596, #20765 ) ;
#24347=FACE_BOUND ( 'NONE', #5559, .T. ) ;
#24390=VECTOR ( 'NONE', #26220, 1000.000000000000114 ) ;
#24397=DIRECTION ( 'NONE',  ( 0.3853207896976533209, -0.9227826878668545785, 0.000000000000000000 ) ) ;
#24413=EDGE_CURVE ( 'NONE', #14963, #3188, #3876, .T. ) ;
#24415=ORIENTED_EDGE ( 'NONE', *, *, #47501, .F. ) ;
#24417=DIRECTION ( 'NONE',  ( 0.02332147558787931590, 0.9997280174009348652, -0.000000000000000000 ) ) ;
#24437=LINE ( 'NONE', #43532, #18418 ) ;
#24463=CARTESIAN_POINT ( 'NONE',  ( -18.24502636017238899, -100.7225776329765665, 5.500000000000000000 ) ) ;
#24475=DIRECTION ( 'NONE',  ( 0.7273375899149793211, -0.6862798483830554463, 0.000000000000000000 ) ) ;
#24487=DIRECTION ( 'NONE',  ( 0.9730327541852497042, -0.2306669878475622604, 0.000000000000000000 ) ) ;
#24517=EDGE_LOOP ( 'NONE', ( #1074, #23622, #44936, #15320 ) ) ;
#24521=VECTOR ( 'NONE', #23858, 1000.000000000000114 ) ;
#24527=ORIENTED_EDGE ( 'NONE', *, *, #27644, .T. ) ;
#24532=DIRECTION ( 'NONE',  ( -0.8774505977381978905, -0.4796670183876304283, 0.000000000000000000 ) ) ;
#24543=LINE ( 'NONE', #2495, #40334 ) ;
#24549=VERTEX_POINT ( 'NONE', #12436 ) ;
#24555=PLANE ( 'NONE',  #45032 ) ;
#24556=VERTEX_POINT ( 'NONE', #5095 ) ;
#24562=DIRECTION ( 'NONE',  ( -0.1276937514489705217, -0.9918136447140101231, 0.000000000000000000 ) ) ;
#24566=CARTESIAN_POINT ( 'NONE',  ( 12.13205353604972991, -140.1820037904669789, -5.500000000000000000 ) ) ;
#24582=VECTOR ( 'NONE', #6890, 1000.000000000000000 ) ;
#24600=ORIENTED_EDGE ( 'NONE', *, *, #1456, .F. ) ;
#24602=EDGE_LOOP ( 'NONE', ( #5141, #23498, #40407, #36124 ) ) ;
#24614=FACE_OUTER_BOUND ( 'NONE', #4011, .T. ) ;
#24625=VECTOR ( 'NONE', #46420, 999.9999999999998863 ) ;
#24629=LINE ( 'NONE', #39573, #4299 ) ;
#24645=ORIENTED_EDGE ( 'NONE', *, *, #37768, .T. ) ;
#24646=ORIENTED_EDGE ( 'NONE', *, *, #1703, .F. ) ;
#24649=VERTEX_POINT ( 'NONE', #31052 ) ;
#24651=DIRECTION ( 'NONE',  ( -0.9966891607226785466, -0.08130631524009969413, 0.000000000000000000 ) ) ;
#24660=EDGE_CURVE ( 'NONE', #38904, #14239, #11953, .T. ) ;
#24663=AXIS2_PLACEMENT_3D ( 'NONE', #26300, #18467, #26540 ) ;
#24686=DIRECTION ( 'NONE',  ( -0.000000000000000000, -0.000000000000000000, 1.000000000000000000 ) ) ;
#24706=ORIENTED_EDGE ( 'NONE', *, *, #26011, .F. ) ;
#24707=ADVANCED_FACE ( 'NONE', ( #47166 ), #13638, .F. ) ;
#24715=ORIENTED_EDGE ( 'NONE', *, *, #27715, .F. ) ;
#24716=CARTESIAN_POINT ( 'NONE',  ( -16.06301359042743115, -102.7814171781257357, 5.500000000000000000 ) ) ;
#24743=DIRECTION ( 'NONE',  ( -0.9781476007338042455, -0.2079116908177664758, 0.000000000000000000 ) ) ;
#24744=CARTESIAN_POINT ( 'NONE',  ( -10.43921258969510824, -98.89258801967538659, 2.500000000000000000 ) ) ;
#24746=DIRECTION ( 'NONE',  ( -0.000000000000000000, -0.000000000000000000, -1.000000000000000000 ) ) ;
#24765=EDGE_LOOP ( 'NONE', ( #36390, #14024, #24009, #9329 ) ) ;
#24766=LINE ( 'NONE', #29399, #11803 ) ;
#24767=EDGE_CURVE ( 'NONE', #43974, #39583, #16835, .T. ) ;
#24771=CARTESIAN_POINT ( 'NONE',  ( 13.36581099891334645, -139.3288669181958710, 2.500000000000000000 ) ) ;
#24776=FACE_BOUND ( 'NONE', #4736, .T. ) ;
#24792=EDGE_LOOP ( 'NONE', ( #24415, #17095, #22175, #1600 ) ) ;
#24793=DIRECTION ( 'NONE',  ( -0.9038112904824846527, 0.4279312458752990711, 0.000000000000000000 ) ) ;
#24795=CARTESIAN_POINT ( 'NONE',  ( 26.47460221209471598, -121.8961639463267090, -5.500000000000000000 ) ) ;
#24807=CARTESIAN_POINT ( 'NONE',  ( -22.53294031248082163, -134.0273518838794757, 5.500000000000000000 ) ) ;
#24824=LINE ( 'NONE', #32420, #29703 ) ;
#24851=FACE_OUTER_BOUND ( 'NONE', #2356, .T. ) ;
#24852=FACE_OUTER_BOUND ( 'NONE', #25165, .T. ) ;
#24866=ORIENTED_EDGE ( 'NONE', *, *, #16677, .T. ) ;
#24870=PLANE ( 'NONE',  #12496 ) ;
#24878=EDGE_LOOP ( 'NONE', ( #40084, #6371, #28680, #2070 ) ) ;
#24879=ORIENTED_EDGE ( 'NONE', *, *, #15541, .T. ) ;
#24897=EDGE_CURVE ( 'NONE', #17292, #38735, #10444, .T. ) ;
#24901=LINE ( 'NONE', #20758, #47798 ) ;
#24908=ORIENTED_EDGE ( 'NONE', *, *, #36844, .F. ) ;
#24909=CARTESIAN_POINT ( 'NONE',  ( 18.80329974962065265, -105.8248132807389084, -5.500000000000000000 ) ) ;
#24916=CARTESIAN_POINT ( 'NONE',  ( -0.8815729230226007074, -93.47222532549339746, -2.500000000000000000 ) ) ;
#24934=CARTESIAN_POINT ( 'NONE',  ( -25.50183398199384754, -112.6408924756582053, 2.500000000000000000 ) ) ;
#24959=CARTESIAN_POINT ( 'NONE',  ( 0.000000000000000000, -120.0000000000000000, -2.500000000000000000 ) ) ;
#24981=ORIENTED_EDGE ( 'NONE', *, *, #4390, .F. ) ;
#24984=DIRECTION ( 'NONE',  ( 0.6516173805718058487, -0.7585478161175724932, 0.000000000000000000 ) ) ;
#24995=LINE ( 'NONE', #18121, #16071 ) ;
#25002=ORIENTED_EDGE ( 'NONE', *, *, #37446, .T. ) ;
#25004=CARTESIAN_POINT ( 'NONE',  ( 6.377742925735834234, -145.7647898336708181, 5.500000000000000000 ) ) ;
#25034=ADVANCED_FACE ( 'NONE', ( #8456 ), #30742, .F. ) ;
#25042=ORIENTED_EDGE ( 'NONE', *, *, #18947, .F. ) ;
#25079=CARTESIAN_POINT ( 'NONE',  ( -23.30023580412278505, -123.4057321492263384, 5.500000000000000000 ) ) ;
#25102=EDGE_CURVE ( 'NONE', #33083, #23423, #42964, .T. ) ;
#25110=VERTEX_POINT ( 'NONE', #47106 ) ;
#25132=DIRECTION ( 'NONE',  ( 1.000000000000000000, 0.000000000000000000, 0.000000000000000000 ) ) ;
#25134=LINE ( 'NONE', #17550, #41563 ) ;
#25135=ORIENTED_EDGE ( 'NONE', *, *, #39034, .F. ) ;
#25143=ADVANCED_FACE ( 'NONE', ( #24347, #31728 ), #31472, .F. ) ;
#25165=EDGE_LOOP ( 'NONE', ( #13275, #28736, #14300, #8485 ) ) ;
#25175=ADVANCED_FACE ( 'NONE', ( #47362 ), #28517, .F. ) ;
#25189=DIRECTION ( 'NONE',  ( -0.7585478161175716050, -0.6516173805718067369, 0.000000000000000000 ) ) ;
#25201=DIRECTION ( 'NONE',  ( -0.2306669878475648139, -0.9730327541852491491, 0.000000000000000000 ) ) ;
#25205=AXIS2_PLACEMENT_3D ( 'NONE', #36687, #3152, #18080 ) ;
#25213=VERTEX_POINT ( 'NONE', #43678 ) ;
#25229=CARTESIAN_POINT ( 'NONE',  ( -89.17737905728745318, -39.70432723693717492, -5.500000000000000000 ) ) ;
#25239=ADVANCED_FACE ( 'NONE', ( #29230 ), #6475, .F. ) ;
#25245=DIRECTION ( 'NONE',  ( -0.7585478161175723821, -0.6516173805718057377, 0.000000000000000000 ) ) ;
#25256=VECTOR ( 'NONE', #10935, 1000.000000000000114 ) ;
#25258=AXIS2_PLACEMENT_3D ( 'NONE', #33446, #45192, #45418 ) ;
#25268=ORIENTED_EDGE ( 'NONE', *, *, #21048, .T. ) ;
#25282=CARTESIAN_POINT ( 'NONE',  ( 8.700667342345820288, -98.11853780484867116, 5.500000000000000000 ) ) ;
#25285=VECTOR ( 'NONE', #15516, 1000.000000000000227 ) ;
#25289=EDGE_LOOP ( 'NONE', ( #30865, #32819, #30851, #43147 ) ) ;
#25299=VECTOR ( 'NONE', #17199, 1000.000000000000000 ) ;
#25310=ORIENTED_EDGE ( 'NONE', *, *, #21619, .F. ) ;
#25319=CARTESIAN_POINT ( 'NONE',  ( 0.000000000000000000, -120.0000000000000000, 5.500000000000000000 ) ) ;
#25328=CARTESIAN_POINT ( 'NONE',  ( 70.53423027509757048, -217.0820393249931044, 5.500000000000000000 ) ) ;
#25344=VECTOR ( 'NONE', #8230, 1000.000000000000114 ) ;
#25345=ORIENTED_EDGE ( 'NONE', *, *, #6629, .T. ) ;
#25348=DIRECTION ( 'NONE',  ( 0.7585478161175706058, 0.6516173805718080692, -0.000000000000000000 ) ) ;
#25350=CARTESIAN_POINT ( 'NONE',  ( -1.233757462863590115, -120.8531368722710795, -2.500000000000000000 ) ) ;
#25361=ORIENTED_EDGE ( 'NONE', *, *, #23473, .F. ) ;
#25365=ORIENTED_EDGE ( 'NONE', *, *, #31985, .F. ) ;
#25390=CARTESIAN_POINT ( 'NONE',  ( 22.94323693612312809, -114.6983135802921083, 5.500000000000000000 ) ) ;
#25401=ORIENTED_EDGE ( 'NONE', *, *, #46087, .T. ) ;
#25408=AXIS2_PLACEMENT_3D ( 'NONE', #46407, #8470, #19469 ) ;
#25410=VECTOR ( 'NONE', #25785, 1000.000000000000000 ) ;
#25429=FACE_OUTER_BOUND ( 'NONE', #24765, .T. ) ;
#25431=ORIENTED_EDGE ( 'NONE', *, *, #16869, .F. ) ;
#25437=LINE ( 'NONE', #47703, #29699 ) ;
#25441=AXIS2_PLACEMENT_3D ( 'NONE', #38750, #27486, #28194 ) ;
#25465=ADVANCED_FACE ( 'NONE', ( #34566 ), #33851, .F. ) ;
#25469=ORIENTED_EDGE ( 'NONE', *, *, #5688, .T. ) ;
#25470=ORIENTED_EDGE ( 'NONE', *, *, #15948, .F. ) ;
#25478=VERTEX_POINT ( 'NONE', #41691 ) ;
#25485=CARTESIAN_POINT ( 'NONE',  ( 8.700667342345820288, -98.11853780484867116, 5.500000000000000000 ) ) ;
#25500=LINE ( 'NONE', #43866, #39923 ) ;
#25506=CIRCLE ( 'NONE', #27882, 35.50000000000000711 ) ;
#25507=CARTESIAN_POINT ( 'NONE',  ( 13.83832728059186046, -142.6495187161941089, 5.500000000000000000 ) ) ;
#25512=FACE_OUTER_BOUND ( 'NONE', #21153, .T. ) ;
#25514=CARTESIAN_POINT ( 'NONE',  ( 2.047646702416564768, -96.54137380445985173, 5.500000000000000000 ) ) ;
#25531=VECTOR ( 'NONE', #21003, 1000.000000000000000 ) ;
#25533=EDGE_LOOP ( 'NONE', ( #31900, #31847, #22448, #24879 ) ) ;
#25555=ORIENTED_EDGE ( 'NONE', *, *, #13677, .T. ) ;
#25559=DIRECTION ( 'NONE',  ( -0.5687579148473765889, 0.8225049752423776450, 0.000000000000000000 ) ) ;
#25561=VERTEX_POINT ( 'NONE', #16470 ) ;
#25573=CYLINDRICAL_SURFACE ( 'NONE', #16072, 32.50000000000000000 ) ;
#25586=DIRECTION ( 'NONE',  ( -0.8541291221503275466, 0.5200609990132993854, 0.000000000000000000 ) ) ;
#25605=CARTESIAN_POINT ( 'NONE',  ( -23.25244084006223133, -132.7111759872722416, -2.500000000000000000 ) ) ;
#25608=DIRECTION ( 'NONE',  ( 0.6862798483830533369, 0.7273375899149812085, 0.000000000000000000 ) ) ;
#25609=DIRECTION ( 'NONE',  ( 0.000000000000000000, 0.000000000000000000, 1.000000000000000000 ) ) ;
#25617=VECTOR ( 'NONE', #22319, 1000.000000000000114 ) ;
#25637=ORIENTED_EDGE ( 'NONE', *, *, #7410, .F. ) ;
#25644=DIRECTION ( 'NONE',  ( 0.7585478161175723821, 0.6516173805718057377, -0.000000000000000000 ) ) ;
#25651=VERTEX_POINT ( 'NONE', #44343 ) ;
#25660=CARTESIAN_POINT ( 'NONE',  ( -23.54415474984308787, -120.4156646670583086, 5.500000000000000000 ) ) ;
#25689=EDGE_CURVE ( 'NONE', #40958, #24649, #18394, .T. ) ;
#25708=CARTESIAN_POINT ( 'NONE',  ( -17.09243336300205129, -103.8724235629982502, 2.500000000000000000 ) ) ;
#25728=EDGE_CURVE ( 'NONE', #19113, #6225, #25971, .T. ) ;
#25730=ORIENTED_EDGE ( 'NONE', *, *, #5428, .T. ) ;
#25732=CARTESIAN_POINT ( 'NONE',  ( -14.87942725330654348, -141.9795960975983178, 5.500000000000000000 ) ) ;
#25746=CARTESIAN_POINT ( 'NONE',  ( 4.348517481000897078, -143.0941636721797465, 2.500000000000000000 ) ) ;
#25748=CARTESIAN_POINT ( 'NONE',  ( -26.53422223201112828, -120.6595836127786043, 5.500000000000000000 ) ) ;
#25754=LINE ( 'NONE', #40229, #33173 ) ;
#25758=DIRECTION ( 'NONE',  ( 0.5687579148473752566, -0.8225049752423786442, 0.000000000000000000 ) ) ;
#25761=EDGE_LOOP ( 'NONE', ( #1956, #26860 ) ) ;
#25767=EDGE_CURVE ( 'NONE', #42694, #43248, #26231, .T. ) ;
#25785=DIRECTION ( 'NONE',  ( 0.9730327541852497042, -0.2306669878475623159, 0.000000000000000000 ) ) ;
#25787=CARTESIAN_POINT ( 'NONE',  ( 0.000000000000000000, -120.0000000000000000, -5.500000000000000000 ) ) ;
#25793=EDGE_CURVE ( 'NONE', #20850, #38904, #12274, .T. ) ;
#25805=LINE ( 'NONE', #28772, #21561 ) ;
#25829=CARTESIAN_POINT ( 'NONE',  ( 3.429551818649054340, -146.3199197248623875, -5.500000000000000000 ) ) ;
#25833=CARTESIAN_POINT ( 'NONE',  ( -1.192633404626841198, -119.0902607174754451, -2.500000000000000000 ) ) ;
#25849=CARTESIAN_POINT ( 'NONE',  ( 0.000000000000000000, -120.0000000000000000, 2.500000000000000000 ) ) ;
#25850=CARTESIAN_POINT ( 'NONE',  ( 15.07208474345548055, -141.7963818439230010, 2.500000000000000000 ) ) ;
#25853=ORIENTED_EDGE ( 'NONE', *, *, #13597, .F. ) ;
#25861=EDGE_CURVE ( 'NONE', #1613, #22152, #19112, .T. ) ;
#25864=VECTOR ( 'NONE', #9787, 1000.000000000000114 ) ;
#25870=PLANE ( 'NONE',  #13815 ) ;
#25874=DIRECTION ( 'NONE',  ( 0.1850432970638656860, -0.9827303690289285187, 0.000000000000000000 ) ) ;
#25885=EDGE_CURVE ( 'NONE', #13231, #37836, #30619, .T. ) ;
#25896=VERTEX_POINT ( 'NONE', #41172 ) ;
#25900=VERTEX_POINT ( 'NONE', #27198 ) ;
#25914=CARTESIAN_POINT ( 'NONE',  ( 0.000000000000000000, 0.000000000000000000, 5.500000000000000000 ) ) ;
#25918=PLANE ( 'NONE',  #39464 ) ;
#25959=DIRECTION ( 'NONE',  ( -0.9038112904824853189, 0.4279312458752976833, 0.000000000000000000 ) ) ;
#25963=DIRECTION ( 'NONE',  ( -0.9730327541852497042, 0.2306669878475622604, 0.000000000000000000 ) ) ;
#25966=ORIENTED_EDGE ( 'NONE', *, *, #32986, .T. ) ;
#25971=LINE ( 'NONE', #10317, #25617 ) ;
#25981=VECTOR ( 'NONE', #35923, 1000.000000000000114 ) ;
#25983=FACE_OUTER_BOUND ( 'NONE', #10904, .T. ) ;
#25990=CARTESIAN_POINT ( 'NONE',  ( -11.59517495878806947, -96.12423995607481686, 5.500000000000000000 ) ) ;
#25991=FACE_OUTER_BOUND ( 'NONE', #25761, .T. ) ;
#26011=EDGE_CURVE ( 'NONE', #43520, #5501, #31851, .T. ) ;
#26015=ORIENTED_EDGE ( 'NONE', *, *, #36477, .F. ) ;
#26035=VECTOR ( 'NONE', #21941, 1000.000000000000000 ) ;
#26038=DIRECTION ( 'NONE',  ( 1.000000000000000000, 0.000000000000000000, 0.000000000000000000 ) ) ;
#26040=CARTESIAN_POINT ( 'NONE',  ( 3.429551818649054340, -146.3199197248623875, 5.500000000000000000 ) ) ;
#26049=CYLINDRICAL_SURFACE ( 'NONE', #24663, 30.50000000000000000 ) ;
#26059=DIRECTION ( 'NONE',  ( 0.5200609990132993854, 0.8541291221503274356, 0.000000000000000000 ) ) ;
#26093=FACE_BOUND ( 'NONE', #36314, .T. ) ;
#26112=ORIENTED_EDGE ( 'NONE', *, *, #18778, .T. ) ;
#26131=VECTOR ( 'NONE', #15380, 1000.000000000000227 ) ;
#26157=ORIENTED_EDGE ( 'NONE', *, *, #43418, .F. ) ;
#26158=CIRCLE ( 'NONE', #1141, 30.50000000000000000 ) ;
#26176=CARTESIAN_POINT ( 'NONE',  ( 0.7195005275814480017, -121.3161758966073052, -2.500000000000000000 ) ) ;
#26179=DIRECTION ( 'NONE',  ( -0.2867529058022035837, 0.9580045777625452175, 0.000000000000000000 ) ) ;
#26185=EDGE_CURVE ( 'NONE', #18083, #5936, #20949, .T. ) ;
#26186=PLANE ( 'NONE',  #33887 ) ;
#26187=LINE ( 'NONE', #34002, #9763 ) ;
#26188=EDGE_CURVE ( 'NONE', #15261, #2795, #7257, .T. ) ;
#26194=CYLINDRICAL_SURFACE ( 'NONE', #36994, 35.50000000000000711 ) ;
#26203=EDGE_CURVE ( 'NONE', #45055, #15896, #44705, .T. ) ;
#26208=ORIENTED_EDGE ( 'NONE', *, *, #34146, .F. ) ;
#26220=DIRECTION ( 'NONE',  ( -0.4279312458753000703, -0.9038112904824842087, 0.000000000000000000 ) ) ;
#26227=DIRECTION ( 'NONE',  ( 0.000000000000000000, -0.000000000000000000, 1.000000000000000000 ) ) ;
#26231=LINE ( 'NONE', #19353, #27171 ) ;
#26232=VERTEX_POINT ( 'NONE', #22190 ) ;
#26251=EDGE_CURVE ( 'NONE', #19471, #40712, #16065, .T. ) ;
#26252=VECTOR ( 'NONE', #29070, 1000.000000000000000 ) ;
#26259=ORIENTED_EDGE ( 'NONE', *, *, #45962, .T. ) ;
#26272=VECTOR ( 'NONE', #18872, 1000.000000000000000 ) ;
#26282=VECTOR ( 'NONE', #24532, 1000.000000000000000 ) ;
#26300=CARTESIAN_POINT ( 'NONE',  ( 0.000000000000000000, -120.0000000000000000, 2.500000000000000000 ) ) ;
#26301=AXIS2_PLACEMENT_3D ( 'NONE', #32246, #28573, #20978 ) ;
#26352=CARTESIAN_POINT ( 'NONE',  ( -11.59517495878806947, -96.12423995607481686, 5.500000000000000000 ) ) ;
#26366=DIRECTION ( 'NONE',  ( 0.9966891607226785466, 0.08130631524009969413, -0.000000000000000000 ) ) ;
#26377=LINE ( 'NONE', #17808, #40979 ) ;
#26400=VECTOR ( 'NONE', #3706, 1000.000000000000000 ) ;
#26401=LINE ( 'NONE', #7783, #8664 ) ;
#26413=EDGE_CURVE ( 'NONE', #25896, #43886, #21406, .T. ) ;
#26423=CARTESIAN_POINT ( 'NONE',  ( 14.59956846177685996, -138.4757300459248484, 5.500000000000000000 ) ) ;
#26433=DIRECTION ( 'NONE',  ( -0.4279312458752977388, -0.9038112904824853189, 0.000000000000000000 ) ) ;
#26435=DIRECTION ( 'NONE',  ( 0.8774505977381978905, 0.4796670183876304283, -0.000000000000000000 ) ) ;
#26439=VECTOR ( 'NONE', #24746, 1000.000000000000000 ) ;
#26458=ORIENTED_EDGE ( 'NONE', *, *, #24660, .T. ) ;
#26465=CARTESIAN_POINT ( 'NONE',  ( 0.000000000000000000, -120.0000000000000000, -2.500000000000000000 ) ) ;
#26471=LINE ( 'NONE', #15459, #1801 ) ;
#26485=LINE ( 'NONE', #45089, #8289 ) ;
#26497=ORIENTED_EDGE ( 'NONE', *, *, #44143, .T. ) ;
#26500=CARTESIAN_POINT ( 'NONE',  ( 12.13205353604972991, -140.1820037904669789, -5.500000000000000000 ) ) ;
#26516=ORIENTED_EDGE ( 'NONE', *, *, #17271, .T. ) ;
#26530=DIRECTION ( 'NONE',  ( -0.000000000000000000, -0.000000000000000000, -1.000000000000000000 ) ) ;
#26540=DIRECTION ( 'NONE',  ( 1.000000000000000000, 0.000000000000000000, 0.000000000000000000 ) ) ;
#26586=DIRECTION ( 'NONE',  ( 0.02332147558787822997, 0.9997280174009349762, 0.000000000000000000 ) ) ;
#26588=DIRECTION ( 'NONE',  ( -0.6064928550163511956, -0.7950889364178798102, 0.000000000000000000 ) ) ;
#26594=EDGE_CURVE ( 'NONE', #43524, #11302, #17965, .T. ) ;
#26612=VECTOR ( 'NONE', #20859, 1000.000000000000114 ) ;
#26634=VECTOR ( 'NONE', #18785, 1000.000000000000000 ) ;
#26651=FACE_OUTER_BOUND ( 'NONE', #5116, .T. ) ;
#26659=FACE_OUTER_BOUND ( 'NONE', #12929, .T. ) ;
#26661=LINE ( 'NONE', #26423, #13616 ) ;
#26667=DIRECTION ( 'NONE',  ( 1.000000000000000000, 0.000000000000000000, 0.000000000000000000 ) ) ;
#26701=CARTESIAN_POINT ( 'NONE',  ( -18.24502636017238899, -100.7225776329765665, -5.500000000000000000 ) ) ;
#26723=LINE ( 'NONE', #42135, #13804 ) ;
#26724=ORIENTED_EDGE ( 'NONE', *, *, #19177, .F. ) ;
#26739=CARTESIAN_POINT ( 'NONE',  ( 6.377742925735834234, -145.7647898336708181, 2.500000000000000000 ) ) ;
#26748=DIRECTION ( 'NONE',  ( -0.9918136447140104561, 0.1276937514489679681, 0.000000000000000000 ) ) ;
#26751=LINE ( 'NONE', #27239, #45764 ) ;
#26768=ORIENTED_EDGE ( 'NONE', *, *, #43863, .T. ) ;
#26803=AXIS2_PLACEMENT_3D ( 'NONE', #35500, #28389, #2209 ) ;
#26814=DIRECTION ( 'NONE',  ( 0.9997280174009348652, -0.02332147558787931590, 0.000000000000000000 ) ) ;
#26839=CARTESIAN_POINT ( 'NONE',  ( 30.50000000000000000, -120.0000000000000000, -5.500000000000000000 ) ) ;
#26842=DIRECTION ( 'NONE',  ( 0.3090169943749573878, -0.9510565162951503115, 0.000000000000000000 ) ) ;
#26858=VECTOR ( 'NONE', #34591, 1000.000000000000000 ) ;
#26860=ORIENTED_EDGE ( 'NONE', *, *, #46361, .F. ) ;
#26875=AXIS2_PLACEMENT_3D ( 'NONE', #22218, #3610, #25874 ) ;
#26896=VECTOR ( 'NONE', #2353, 1000.000000000000000 ) ;
#26916=( NAMED_UNIT ( * ) PLANE_ANGLE_UNIT ( ) SI_UNIT ( $, .RADIAN. ) );
#26920=ORIENTED_EDGE ( 'NONE', *, *, #9230, .T. ) ;
#26943=EDGE_CURVE ( 'NONE', #5822, #30085, #33340, .T. ) ;
#26944=CARTESIAN_POINT ( 'NONE',  ( 12.50000000000000000, -107.5000000000000000, 2.500000000000000000 ) ) ;
#26951=DIRECTION ( 'NONE',  ( -0.9038112904824853189, 0.4279312458752976833, 0.000000000000000000 ) ) ;
#26967=DIRECTION ( 'NONE',  ( -0.000000000000000000, -0.000000000000000000, -1.000000000000000000 ) ) ;
#26968=DIRECTION ( 'NONE',  ( -0.000000000000000000, -0.000000000000000000, -1.000000000000000000 ) ) ;
#26969=CARTESIAN_POINT ( 'NONE',  ( 12.69589495141918611, -96.69089767102708777, 5.500000000000000000 ) ) ;
#26978=PLANE ( 'NONE',  #7524 ) ;
#26986=DIRECTION ( 'NONE',  ( -0.000000000000000000, -0.000000000000000000, -1.000000000000000000 ) ) ;
#26989=VERTEX_POINT ( 'NONE', #21826 ) ;
#26996=DIRECTION ( 'NONE',  ( -0.2867529058022021404, 0.9580045777625456616, 0.000000000000000000 ) ) ;
#27001=VECTOR ( 'NONE', #38253, 1000.000000000000114 ) ;
#27031=CARTESIAN_POINT ( 'NONE',  ( -18.12185313557660038, -104.9634299478706794, 2.500000000000000000 ) ) ;
#27034=DIRECTION ( 'NONE',  ( -0.000000000000000000, -0.000000000000000000, -1.000000000000000000 ) ) ;
#27053=ORIENTED_EDGE ( 'NONE', *, *, #27901, .F. ) ;
#27055=ORIENTED_EDGE ( 'NONE', *, *, #46135, .F. ) ;
#27085=DIRECTION ( 'NONE',  ( 0.08130631524010117905, -0.9966891607226784355, 0.000000000000000000 ) ) ;
#27086=DIRECTION ( 'NONE',  ( 0.5200609990132993854, 0.8541291221503275466, 0.000000000000000000 ) ) ;
#27094=LINE ( 'NONE', #7265, #21240 ) ;
#27101=PLANE ( 'NONE',  #31095 ) ;
#27114=ORIENTED_EDGE ( 'NONE', *, *, #6674, .F. ) ;
#27117=LINE ( 'NONE', #35400, #4631 ) ;
#27123=VERTEX_POINT ( 'NONE', #31125 ) ;
#27132=ORIENTED_EDGE ( 'NONE', *, *, #2960, .F. ) ;
#27133=ORIENTED_EDGE ( 'NONE', *, *, #12839, .T. ) ;
#27171=VECTOR ( 'NONE', #11308, 1000.000000000000000 ) ;
#27173=ORIENTED_EDGE ( 'NONE', *, *, #30546, .F. ) ;
#27174=VECTOR ( 'NONE', #3348, 1000.000000000000114 ) ;
#27187=EDGE_CURVE ( 'NONE', #17554, #25213, #38457, .T. ) ;
#27198=CARTESIAN_POINT ( 'NONE',  ( -14.87942725330654348, -141.9795960975983178, -2.500000000000000000 ) ) ;
#27204=LINE ( 'NONE', #45809, #15950 ) ;
#27210=ADVANCED_FACE ( 'NONE', ( #16664 ), #32087, .F. ) ;
#27215=DIRECTION ( 'NONE',  ( -0.000000000000000000, -0.000000000000000000, -1.000000000000000000 ) ) ;
#27222=VECTOR ( 'NONE', #44217, 1000.000000000000114 ) ;
#27229=DIRECTION ( 'NONE',  ( -0.9580045777625456616, -0.2867529058022021404, 0.000000000000000000 ) ) ;
#27239=CARTESIAN_POINT ( 'NONE',  ( -23.42219527698293646, -121.9106984081423803, -2.500000000000000000 ) ) ;
#27244=ADVANCED_FACE ( 'NONE', ( #38717 ), #1992, .F. ) ;
#27246=ADVANCED_FACE ( 'NONE', ( #28161 ), #46285, .T. ) ;
#27251=CARTESIAN_POINT ( 'NONE',  ( -6.880223345695647197, -142.5202692415819854, 2.500000000000000000 ) ) ;
#27253=EDGE_LOOP ( 'NONE', ( #41208, #27613, #13610, #10006 ) ) ;
#27261=DIRECTION ( 'NONE',  ( 0.2867529058022035837, -0.9580045777625452175, 0.000000000000000000 ) ) ;
#27352=DIRECTION ( 'NONE',  ( -0.9918136447140100120, 0.1276937514489704939, 0.000000000000000000 ) ) ;
#27355=ORIENTED_EDGE ( 'NONE', *, *, #12073, .T. ) ;
#27356=EDGE_CURVE ( 'NONE', #38735, #46006, #22005, .T. ) ;
#27360=DIRECTION ( 'NONE',  ( 0.8774505977381978905, 0.4796670183876304283, 0.000000000000000000 ) ) ;
#27368=LINE ( 'NONE', #42544, #42090 ) ;
#27384=DIRECTION ( 'NONE',  ( 1.000000000000000000, 0.000000000000000000, 0.000000000000000000 ) ) ;
#27396=VECTOR ( 'NONE', #38205, 1000.000000000000000 ) ;
#27400=ORIENTED_EDGE ( 'NONE', *, *, #1759, .T. ) ;
#27408=CARTESIAN_POINT ( 'NONE',  ( 32.50000000000000000, -120.0000000000000000, -2.500000000000000000 ) ) ;
#27410=ORIENTED_EDGE ( 'NONE', *, *, #43763, .T. ) ;
#27421=EDGE_CURVE ( 'NONE', #23846, #19505, #25437, .T. ) ;
#27444=DIRECTION ( 'NONE',  ( 0.6064928550163524168, 0.7950889364178788110, 0.000000000000000000 ) ) ;
#27462=ORIENTED_EDGE ( 'NONE', *, *, #6156, .T. ) ;
#27468=MECHANICAL_DESIGN_GEOMETRIC_PRESENTATION_REPRESENTATION('',(#5479),#18731);
#27471=EDGE_CURVE ( 'NONE', #16641, #10301, #4624, .T. ) ;
#27486=DIRECTION ( 'NONE',  ( 0.2867529058022011967, -0.9580045777625459946, 0.000000000000000000 ) ) ;
#27491=DIRECTION ( 'NONE',  ( 0.2867529058022011967, -0.9580045777625459946, 0.000000000000000000 ) ) ;
#27500=ORIENTED_EDGE ( 'NONE', *, *, #32356, .F. ) ;
#27501=VECTOR ( 'NONE', #26530, 1000.000000000000000 ) ;
#27506=EDGE_LOOP ( 'NONE', ( #39170, #28079, #28850, #8674 ) ) ;
#27522=EDGE_CURVE ( 'NONE', #45508, #18661, #48437, .T. ) ;
#27539=ORIENTED_EDGE ( 'NONE', *, *, #44906, .F. ) ;
#27567=DIRECTION ( 'NONE',  ( 0.7950889364178798102, -0.6064928550163511956, 0.000000000000000000 ) ) ;
#27570=LINE ( 'NONE', #42500, #40487 ) ;
#27572=LINE ( 'NONE', #39071, #38062 ) ;
#27575=EDGE_CURVE ( 'NONE', #5156, #28753, #37921, .T. ) ;
#27601=PLANE ( 'NONE',  #24328 ) ;
#27608=VERTEX_POINT ( 'NONE', #25829 ) ;
#27612=EDGE_CURVE ( 'NONE', #6148, #28620, #44681, .T. ) ;
#27613=ORIENTED_EDGE ( 'NONE', *, *, #20611, .T. ) ;
#27617=FACE_OUTER_BOUND ( 'NONE', #46193, .T. ) ;
#27624=VECTOR ( 'NONE', #34164, 1000.000000000000000 ) ;
#27630=CARTESIAN_POINT ( 'NONE',  ( -10.43921258969510824, -98.89258801967538659, -5.500000000000000000 ) ) ;
#27636=ORIENTED_EDGE ( 'NONE', *, *, #42394, .T. ) ;
#27644=EDGE_CURVE ( 'NONE', #10301, #43899, #14837, .T. ) ;
#27656=ORIENTED_EDGE ( 'NONE', *, *, #43763, .F. ) ;
#27662=EDGE_LOOP ( 'NONE', ( #4450, #22901, #32829, #26768 ) ) ;
#27667=VECTOR ( 'NONE', #13744, 1000.000000000000000 ) ;
#27675=DIRECTION ( 'NONE',  ( -0.000000000000000000, -0.000000000000000000, 1.000000000000000000 ) ) ;
#27695=DIRECTION ( 'NONE',  ( 0.08130631524010117905, -0.9966891607226784355, 0.000000000000000000 ) ) ;
#27715=EDGE_CURVE ( 'NONE', #5563, #27123, #47626, .T. ) ;
#27722=ORIENTED_EDGE ( 'NONE', *, *, #48241, .F. ) ;
#27728=VECTOR ( 'NONE', #17997, 1000.000000000000114 ) ;
#27732=ORIENTED_EDGE ( 'NONE', *, *, #35252, .F. ) ;
#27744=EDGE_LOOP ( 'NONE', ( #6531, #2193, #9573, #39207 ) ) ;
#27764=FACE_OUTER_BOUND ( 'NONE', #42172, .T. ) ;
#27782=ORIENTED_EDGE ( 'NONE', *, *, #8553, .F. ) ;
#27793=VECTOR ( 'NONE', #14197, 1000.000000000000000 ) ;
#27820=VECTOR ( 'NONE', #19391, 1000.000000000000114 ) ;
#27822=EDGE_LOOP ( 'NONE', ( #2538, #3677, #16349, #14711 ) ) ;
#27836=DIRECTION ( 'NONE',  ( -0.000000000000000000, -0.000000000000000000, 1.000000000000000000 ) ) ;
#27838=VERTEX_POINT ( 'NONE', #42218 ) ;
#27846=EDGE_LOOP ( 'NONE', ( #20989, #32768, #31657, #13871 ) ) ;
#27856=AXIS2_PLACEMENT_3D ( 'NONE', #45876, #12344, #23577 ) ;
#27882=AXIS2_PLACEMENT_3D ( 'NONE', #30829, #45754, #26667 ) ;
#27901=EDGE_CURVE ( 'NONE', #5822, #23903, #47098, .T. ) ;
#27914=CARTESIAN_POINT ( 'NONE',  ( -24.50849501662245800, -109.8101191361138831, 5.500000000000000000 ) ) ;
#27927=CARTESIAN_POINT ( 'NONE',  ( -23.97194136764370498, -131.3950000906648938, 5.500000000000000000 ) ) ;
#27942=PLANE ( 'NONE',  #1124 ) ;
#27945=CARTESIAN_POINT ( 'NONE',  ( 0.000000000000000000, -120.0000000000000000, 2.500000000000000000 ) ) ;
#27972=ORIENTED_EDGE ( 'NONE', *, *, #18523, .F. ) ;
#27977=LINE ( 'NONE', #23807, #13434 ) ;
#27982=DIRECTION ( 'NONE',  ( 1.000000000000000000, 0.000000000000000000, 0.000000000000000000 ) ) ;
#28015=ADVANCED_FACE ( 'NONE', ( #21141 ), #1356, .F. ) ;
#28022=LINE ( 'NONE', #46368, #24521 ) ;
#28026=CARTESIAN_POINT ( 'NONE',  ( 12.69589495141918611, -96.69089767102708777, 5.500000000000000000 ) ) ;
#28033=CARTESIAN_POINT ( 'NONE',  ( 11.41210121379328335, -99.40233154247455616, -5.500000000000000000 ) ) ;
#28037=ORIENTED_EDGE ( 'NONE', *, *, #3950, .F. ) ;
#28045=DIRECTION ( 'NONE',  ( -0.000000000000000000, -0.000000000000000000, -1.000000000000000000 ) ) ;
#28050=DIRECTION ( 'NONE',  ( -0.9966891607226785466, -0.08130631524010122069, 0.000000000000000000 ) ) ;
#28055=CARTESIAN_POINT ( 'NONE',  ( -13.05994868825747446, -139.5943292883446532, 5.500000000000000000 ) ) ;
#28056=CARTESIAN_POINT ( 'NONE',  ( -4.653126046682595884, -146.1313684676804314, 5.500000000000000000 ) ) ;
#28059=LINE ( 'NONE', #25514, #3751 ) ;
#28061=LINE ( 'NONE', #42989, #6577 ) ;
#28062=VERTEX_POINT ( 'NONE', #11610 ) ;
#28069=EDGE_CURVE ( 'NONE', #21809, #8377, #18926, .T. ) ;
#28078=VECTOR ( 'NONE', #12419, 1000.000000000000114 ) ;
#28079=ORIENTED_EDGE ( 'NONE', *, *, #2298, .T. ) ;
#28083=EDGE_CURVE ( 'NONE', #32049, #29568, #37547, .T. ) ;
#28101=ORIENTED_EDGE ( 'NONE', *, *, #21248, .F. ) ;
#28111=VERTEX_POINT ( 'NONE', #45368 ) ;
#28124=CARTESIAN_POINT ( 'NONE',  ( -1.384174031800281979, -120.5779811845464735, 2.500000000000000000 ) ) ;
#28126=EDGE_CURVE ( 'NONE', #46006, #6288, #33867, .T. ) ;
#28128=PLANE ( 'NONE',  #42216 ) ;
#28139=EDGE_CURVE ( 'NONE', #11421, #21809, #3533, .T. ) ;
#28154=ORIENTED_EDGE ( 'NONE', *, *, #42836, .T. ) ;
#28158=DIRECTION ( 'NONE',  ( 0.7950889364178788110, -0.6064928550163524168, 0.000000000000000000 ) ) ;
#28161=FACE_OUTER_BOUND ( 'NONE', #32225, .T. ) ;
#28172=ORIENTED_EDGE ( 'NONE', *, *, #9884, .T. ) ;
#28189=ORIENTED_EDGE ( 'NONE', *, *, #3804, .F. ) ;
#28194=DIRECTION ( 'NONE',  ( 0.9580045777625458836, 0.2867529058022011412, 0.000000000000000000 ) ) ;
#28198=FACE_OUTER_BOUND ( 'NONE', #21747, .T. ) ;
#28199=LINE ( 'NONE', #40434, #24582 ) ;
#28219=CARTESIAN_POINT ( 'NONE',  ( 3.429551818649054340, -146.3199197248623875, 2.500000000000000000 ) ) ;
#28227=LINE ( 'NONE', #1567, #40426 ) ;
#28234=VERTEX_POINT ( 'NONE', #19413 ) ;
#28238=CARTESIAN_POINT ( 'NONE',  ( -4.653126046682595884, -146.1313684676804314, 5.500000000000000000 ) ) ;
#28247=EDGE_CURVE ( 'NONE', #46719, #9902, #42685, .T. ) ;
#28252=DIRECTION ( 'NONE',  ( -0.6064928550163533050, -0.7950889364178781449, 0.000000000000000000 ) ) ;
#28255=VECTOR ( 'NONE', #45061, 1000.000000000000114 ) ;
#28274=CARTESIAN_POINT ( 'NONE',  ( 24.95699195200416654, -110.9640411295978595, 5.500000000000000000 ) ) ;
#28303=ORIENTED_EDGE ( 'NONE', *, *, #23480, .T. ) ;
#28317=VERTEX_POINT ( 'NONE', #47316 ) ;
#28354=EDGE_CURVE ( 'NONE', #43524, #33083, #36286, .T. ) ;
#28358=VERTEX_POINT ( 'NONE', #28219 ) ;
#28364=ORIENTED_EDGE ( 'NONE', *, *, #28636, .T. ) ;
#28389=DIRECTION ( 'NONE',  ( 0.000000000000000000, 0.000000000000000000, 1.000000000000000000 ) ) ;
#28400=CARTESIAN_POINT ( 'NONE',  ( 119.3426274441929280, -132.5434155921172419, -5.500000000000000000 ) ) ;
#28424=EDGE_CURVE ( 'NONE', #43507, #19471, #17188, .T. ) ;
#28436=CARTESIAN_POINT ( 'NONE',  ( -18.12185313557659683, -104.9634299478706794, -2.500000000000000000 ) ) ;
#28440=VERTEX_POINT ( 'NONE', #24795 ) ;
#28458=LINE ( 'NONE', #5962, #29780 ) ;
#28459=ORIENTED_EDGE ( 'NONE', *, *, #28354, .T. ) ;
#28484=ORIENTED_EDGE ( 'NONE', *, *, #43811, .T. ) ;
#28499=AXIS2_PLACEMENT_3D ( 'NONE', #40772, #7491, #40534 ) ;
#28505=VECTOR ( 'NONE', #1026, 1000.000000000000000 ) ;
#28507=EDGE_LOOP ( 'NONE', ( #44194, #8445, #8269, #29123 ) ) ;
#28510=VERTEX_POINT ( 'NONE', #37730 ) ;
#28515=ADVANCED_FACE ( 'NONE', ( #25983 ), #22067, .F. ) ;
#28517=PLANE ( 'NONE',  #14638 ) ;
#28518=ORIENTED_EDGE ( 'NONE', *, *, #17472, .T. ) ;
#28520=LINE ( 'NONE', #17483, #15272 ) ;
#28529=CARTESIAN_POINT ( 'NONE',  ( -35.50000000000000711, -120.0000000000000000, 5.500000000000000000 ) ) ;
#28562=EDGE_CURVE ( 'NONE', #41259, #23903, #47764, .T. ) ;
#28564=ORIENTED_EDGE ( 'NONE', *, *, #45513, .F. ) ;
#28573=DIRECTION ( 'NONE',  ( 0.000000000000000000, 0.000000000000000000, 1.000000000000000000 ) ) ;
#28578=CARTESIAN_POINT ( 'NONE',  ( 12.50000000000000000, -107.5000000000000000, -2.500000000000000000 ) ) ;
#28603=ORIENTED_EDGE ( 'NONE', *, *, #37957, .T. ) ;
#28607=CARTESIAN_POINT ( 'NONE',  ( -7.670864526094547386, -97.73662565058241114, -2.500000000000000000 ) ) ;
#28619=VERTEX_POINT ( 'NONE', #19837 ) ;
#28620=VERTEX_POINT ( 'NONE', #38459 ) ;
#28624=EDGE_CURVE ( 'NONE', #39725, #4261, #1502, .T. ) ;
#28630=DIRECTION ( 'NONE',  ( -0.5687579148473752566, 0.8225049752423786442, 0.000000000000000000 ) ) ;
#28636=EDGE_CURVE ( 'NONE', #45971, #47873, #16196, .T. ) ;
#28650=DIRECTION ( 'NONE',  ( -0.000000000000000000, -0.000000000000000000, -1.000000000000000000 ) ) ;
#28671=ORIENTED_EDGE ( 'NONE', *, *, #34576, .F. ) ;
#28675=PLANE ( 'NONE',  #42190 ) ;
#28680=ORIENTED_EDGE ( 'NONE', *, *, #14208, .T. ) ;
#28687=ORIENTED_EDGE ( 'NONE', *, *, #23480, .F. ) ;
#28695=FACE_OUTER_BOUND ( 'NONE', #12905, .T. ) ;
#28731=CARTESIAN_POINT ( 'NONE',  ( 26.47460221209471598, -121.8961639463267090, 5.500000000000000000 ) ) ;
#28735=EDGE_CURVE ( 'NONE', #28861, #11806, #32943, .T. ) ;
#28736=ORIENTED_EDGE ( 'NONE', *, *, #47501, .T. ) ;
#28752=CARTESIAN_POINT ( 'NONE',  ( -7.572224309238338336, -145.4393675041377492, 5.500000000000000000 ) ) ;
#28753=VERTEX_POINT ( 'NONE', #35260 ) ;
#28772=CARTESIAN_POINT ( 'NONE',  ( -1.192633404626841198, -119.0902607174754451, 2.500000000000000000 ) ) ;
#28791=VERTEX_POINT ( 'NONE', #46536 ) ;
#28801=CARTESIAN_POINT ( 'NONE',  ( 11.41210121379328335, -99.40233154247455616, -5.500000000000000000 ) ) ;
#28814=SURFACE_STYLE_USAGE ( .BOTH. , #43744 ) ;
#28824=DIRECTION ( 'NONE',  ( -0.000000000000000000, -0.000000000000000000, 1.000000000000000000 ) ) ;
#28825=COLOUR_RGB ( '', 0.08235294, 0.09019608, 0.10196078) ;
#28826=DIRECTION ( 'NONE',  ( 0.02332147558787822997, 0.9997280174009349762, 0.000000000000000000 ) ) ;
#28834=ADVANCED_FACE ( 'NONE', ( #40086 ), #29061, .F. ) ;
#28850=ORIENTED_EDGE ( 'NONE', *, *, #7948, .T. ) ;
#28861=VERTEX_POINT ( 'NONE', #41300 ) ;
#28874=EDGE_CURVE ( 'NONE', #30819, #7858, #30760, .T. ) ;
#28895=AXIS2_PLACEMENT_3D ( 'NONE', #48294, #29934, #309 ) ;
#28913=DIRECTION ( 'NONE',  ( 0.000000000000000000, 0.000000000000000000, 1.000000000000000000 ) ) ;
#28951=AXIS2_PLACEMENT_3D ( 'NONE', #38703, #27675, #17354 ) ;
#28952=VERTEX_POINT ( 'NONE', #26839 ) ;
#28958=EDGE_CURVE ( 'NONE', #3684, #11421, #27094, .T. ) ;
#28968=CIRCLE ( 'NONE', #18030, 30.50000000000000000 ) ;
#28979=DIRECTION ( 'NONE',  ( -0.5200609990133016058, -0.8541291221503261033, 0.000000000000000000 ) ) ;
#29000=LINE ( 'NONE', #48329, #459 ) ;
#29003=CARTESIAN_POINT ( 'NONE',  ( -10.43921258969510824, -98.89258801967538659, -5.500000000000000000 ) ) ;
#29024=DIRECTION ( 'NONE',  ( 0.9730327541852497042, -0.2306669878475622604, 0.000000000000000000 ) ) ;
#29029=DIRECTION ( 'NONE',  ( 0.2306669878475647861, 0.9730327541852491491, 0.000000000000000000 ) ) ;
#29032=DIRECTION ( 'NONE',  ( 0.1850432970638667407, -0.9827303690289282967, 0.000000000000000000 ) ) ;
#29042=ORIENTED_EDGE ( 'NONE', *, *, #17802, .T. ) ;
#29047=ORIENTED_EDGE ( 'NONE', *, *, #12906, .T. ) ;
#29059=CARTESIAN_POINT ( 'NONE',  ( -22.53294031248082163, -134.0273518838794757, -5.500000000000000000 ) ) ;
#29061=PLANE ( 'NONE',  #44686 ) ;
#29066=ADVANCED_FACE ( 'NONE', ( #8476 ), #35635, .F. ) ;
#29070=DIRECTION ( 'NONE',  ( -0.000000000000000000, -0.000000000000000000, -1.000000000000000000 ) ) ;
#29073=DIRECTION ( 'NONE',  ( -0.6862798483830544471, -0.7273375899149802093, 0.000000000000000000 ) ) ;
#29079=DIRECTION ( 'NONE',  ( -0.2867529058022035837, 0.9580045777625452175, 0.000000000000000000 ) ) ;
#29100=VERTEX_POINT ( 'NONE', #1621 ) ;
#29118=ADVANCED_FACE ( 'NONE', ( #47597 ), #40512, .T. ) ;
#29120=LINE ( 'NONE', #33032, #46470 ) ;
#29123=ORIENTED_EDGE ( 'NONE', *, *, #26943, .T. ) ;
#29136=ORIENTED_EDGE ( 'NONE', *, *, #25885, .T. ) ;
#29141=VECTOR ( 'NONE', #41301, 1000.000000000000114 ) ;
#29163=ORIENTED_EDGE ( 'NONE', *, *, #33819, .F. ) ;
#29166=DIRECTION ( 'NONE',  ( -0.9966891607226786576, -0.08130631524009861166, 0.000000000000000000 ) ) ;
#29171=ADVANCED_FACE ( 'NONE', ( #24851 ), #6261, .F. ) ;
#29175=DIRECTION ( 'NONE',  ( 0.000000000000000000, -0.000000000000000000, 1.000000000000000000 ) ) ;
#29185=EDGE_CURVE ( 'NONE', #21061, #10970, #12702, .T. ) ;
#29186=CARTESIAN_POINT ( 'NONE',  ( -119.3426274441927433, -132.5434155921188619, -5.500000000000000000 ) ) ;
#29194=PLANE ( 'NONE',  #15983 ) ;
#29230=FACE_OUTER_BOUND ( 'NONE', #10762, .T. ) ;
#29233=VECTOR ( 'NONE', #473, 1000.000000000000000 ) ;
#29248=ORIENTED_EDGE ( 'NONE', *, *, #38670, .T. ) ;
#29257=ORIENTED_EDGE ( 'NONE', *, *, #19320, .T. ) ;
#29259=LINE ( 'NONE', #22146, #37123 ) ;
#29260=VECTOR ( 'NONE', #6413, 1000.000000000000000 ) ;
#29276=LINE ( 'NONE', #14102, #7384 ) ;
#29277=CARTESIAN_POINT ( 'NONE',  ( -0.8815729230226008184, -93.47222532549339746, 5.500000000000000000 ) ) ;
#29306=DIRECTION ( 'NONE',  ( -0.000000000000000000, -0.000000000000000000, -1.000000000000000000 ) ) ;
#29349=CARTESIAN_POINT ( 'NONE',  ( 0.000000000000000000, -120.0000000000000000, -5.500000000000000000 ) ) ;
#29366=CARTESIAN_POINT ( 'NONE',  ( 19.29194287201271862, -133.5026271600380880, 5.500000000000000000 ) ) ;
#29367=LINE ( 'NONE', #212, #33783 ) ;
#29369=FACE_OUTER_BOUND ( 'NONE', #19286, .T. ) ;
#29373=EDGE_LOOP ( 'NONE', ( #12474, #12007, #8800, #37746 ) ) ;
#29385=SHAPE_REPRESENTATION ( 'Sliding Dog Clutch Collar', ( #11636 ), #10062 ) ;
#29389=ORIENTED_EDGE ( 'NONE', *, *, #18523, .T. ) ;
#29393=EDGE_CURVE ( 'NONE', #3571, #44934, #9150, .T. ) ;
#29399=CARTESIAN_POINT ( 'NONE',  ( 35.50000000000000711, -120.0000000000000000, 2.500000000000000000 ) ) ;
#29408=ORIENTED_EDGE ( 'NONE', *, *, #47320, .F. ) ;
#29413=CARTESIAN_POINT ( 'NONE',  ( -3.961125083139900749, -143.2122702051246677, -5.500000000000000000 ) ) ;
#29424=ORIENTED_EDGE ( 'NONE', *, *, #11070, .F. ) ;
#29439=FACE_BOUND ( 'NONE', #46417, .T. ) ;
#29443=ORIENTED_EDGE ( 'NONE', *, *, #46913, .T. ) ;
#29444=VECTOR ( 'NONE', #6013, 1000.000000000000000 ) ;
#29461=DIRECTION ( 'NONE',  ( -0.000000000000000000, -0.000000000000000000, 1.000000000000000000 ) ) ;
#29471=EDGE_LOOP ( 'NONE', ( #42837, #24646, #4139, #47827 ) ) ;
#29481=CARTESIAN_POINT ( 'NONE',  ( 23.49916127795269460, -121.5130826919798039, 5.500000000000000000 ) ) ;
#29485=DIRECTION ( 'NONE',  ( 0.2306669878475647861, 0.9730327541852491491, 0.000000000000000000 ) ) ;
#29499=DIRECTION ( 'NONE',  ( -1.000000000000000000, 0.000000000000000000, 0.000000000000000000 ) ) ;
#29507=EDGE_LOOP ( 'NONE', ( #38363, #9956, #45956, #4577 ) ) ;
#29528=CARTESIAN_POINT ( 'NONE',  ( -23.54415474984308787, -120.4156646670583086, -5.500000000000000000 ) ) ;
#29548=DIRECTION ( 'NONE',  ( 1.000000000000000000, 0.000000000000000000, 0.000000000000000000 ) ) ;
#29550=VECTOR ( 'NONE', #32941, 1000.000000000000114 ) ;
#29553=ADVANCED_FACE ( 'NONE', ( #25512 ), #13541, .F. ) ;
#29564=ORIENTED_EDGE ( 'NONE', *, *, #25861, .T. ) ;
#29568=VERTEX_POINT ( 'NONE', #24566 ) ;
#29571=FACE_OUTER_BOUND ( 'NONE', #44322, .T. ) ;
#29577=DIRECTION ( 'NONE',  ( -0.5200609990133016058, -0.8541291221503261033, 0.000000000000000000 ) ) ;
#29578=EDGE_LOOP ( 'NONE', ( #17904, #28484, #23185, #6474 ) ) ;
#29594=VERTEX_POINT ( 'NONE', #2510 ) ;
#29596=PLANE ( 'NONE',  #41004 ) ;
#29606=EDGE_CURVE ( 'NONE', #44547, #25900, #35816, .T. ) ;
#29613=VERTEX_POINT ( 'NONE', #21358 ) ;
#29626=ORIENTED_EDGE ( 'NONE', *, *, #42394, .F. ) ;
#29628=CARTESIAN_POINT ( 'NONE',  ( 25.81725066941077529, -113.8380548628854854, 5.500000000000000000 ) ) ;
#29646=CARTESIAN_POINT ( 'NONE',  ( 0.000000000000000000, -89.50000000000000000, -5.500000000000000000 ) ) ;
#29648=DIRECTION ( 'NONE',  ( -0.000000000000000000, -0.000000000000000000, -1.000000000000000000 ) ) ;
#29655=LINE ( 'NONE', #17907, #43305 ) ;
#29660=DIRECTION ( 'NONE',  ( 0.9038112904824853189, -0.4279312458752977388, 0.000000000000000000 ) ) ;
#29663=DIRECTION ( 'NONE',  ( 0.02332147558787671729, 0.9997280174009349762, -0.000000000000000000 ) ) ;
#29670=CARTESIAN_POINT ( 'NONE',  ( 2.874421927457452952, -143.3717286177755739, 2.500000000000000000 ) ) ;
#29671=DIRECTION ( 'NONE',  ( -0.000000000000000000, -0.000000000000000000, -1.000000000000000000 ) ) ;
#29672=EDGE_CURVE ( 'NONE', #21021, #21809, #3727, .T. ) ;
#29675=EDGE_LOOP ( 'NONE', ( #26112, #44209 ) ) ;
#29698=LINE ( 'NONE', #44636, #9507 ) ;
#29699=VECTOR ( 'NONE', #18088, 1000.000000000000000 ) ;
#29703=VECTOR ( 'NONE', #36555, 1000.000000000000114 ) ;
#29724=EDGE_CURVE ( 'NONE', #35358, #10091, #34062, .T. ) ;
#29730=LINE ( 'NONE', #44663, #33409 ) ;
#29733=EDGE_CURVE ( 'NONE', #13936, #42659, #22811, .T. ) ;
#29742=EDGE_LOOP ( 'NONE', ( #30859, #14896, #28564, #40430 ) ) ;
#29757=LINE ( 'NONE', #11166, #31166 ) ;
#29760=ORIENTED_EDGE ( 'NONE', *, *, #555, .F. ) ;
#29772=DIRECTION ( 'NONE',  ( -0.000000000000000000, -0.000000000000000000, 1.000000000000000000 ) ) ;
#29780=VECTOR ( 'NONE', #25245, 1000.000000000000114 ) ;
#29785=ADVANCED_FACE ( 'NONE', ( #29439, #25991 ), #30172, .F. ) ;
#29789=PLANE ( 'NONE',  #7994 ) ;
#29794=CARTESIAN_POINT ( 'NONE',  ( -10.43921258969510824, -98.89258801967538659, 5.500000000000000000 ) ) ;
#29809=VERTEX_POINT ( 'NONE', #29911 ) ;
#29811=CARTESIAN_POINT ( 'NONE',  ( 19.29194287201271862, -133.5026271600380880, 5.500000000000000000 ) ) ;
#29842=CARTESIAN_POINT ( 'NONE',  ( 22.08297821871651934, -111.8242998470044540, 5.500000000000000000 ) ) ;
#29851=VECTOR ( 'NONE', #27034, 1000.000000000000000 ) ;
#29855=EDGE_CURVE ( 'NONE', #47761, #21860, #13019, .T. ) ;
#29879=ORIENTED_EDGE ( 'NONE', *, *, #32647, .F. ) ;
#29891=EDGE_LOOP ( 'NONE', ( #7198, #5030, #46792, #34851 ) ) ;
#29894=PLANE ( 'NONE',  #21479 ) ;
#29911=CARTESIAN_POINT ( 'NONE',  ( 24.95699195200417364, -110.9640411295978595, -2.500000000000000000 ) ) ;
#29913=FACE_OUTER_BOUND ( 'NONE', #4780, .T. ) ;
#29924=VECTOR ( 'NONE', #21213, 1000.000000000000000 ) ;
#29934=DIRECTION ( 'NONE',  ( 0.4796670183876304283, -0.8774505977381978905, 0.000000000000000000 ) ) ;
#29935=FACE_OUTER_BOUND ( 'NONE', #14544, .T. ) ;
#29936=VERTEX_POINT ( 'NONE', #8120 ) ;
#29948=VERTEX_POINT ( 'NONE', #24744 ) ;
#29980=ADVANCED_FACE ( 'NONE', ( #6140 ), #43102, .F. ) ;
#29987=AXIS2_PLACEMENT_3D ( 'NONE', #38514, #19411, #4979 ) ;
#30001=ORIENTED_EDGE ( 'NONE', *, *, #24413, .F. ) ;
#30031=PLANE ( 'NONE',  #36657 ) ;
#30054=AXIS2_PLACEMENT_3D ( 'NONE', #22337, #29663, #31078 ) ;
#30068=CARTESIAN_POINT ( 'NONE',  ( 20.85212586905262100, -130.9402397935870965, -5.500000000000000000 ) ) ;
#30070=FACE_OUTER_BOUND ( 'NONE', #40094, .T. ) ;
#30085=VERTEX_POINT ( 'NONE', #47961 ) ;
#30087=PLANE ( 'NONE',  #35274 ) ;
#30097=CARTESIAN_POINT ( 'NONE',  ( -30.50000000000000000, -120.0000000000000000, 5.500000000000000888 ) ) ;
#30108=DIRECTION ( 'NONE',  ( -0.000000000000000000, -0.000000000000000000, -1.000000000000000000 ) ) ;
#30110=EDGE_LOOP ( 'NONE', ( #47752, #30980 ) ) ;
#30129=VECTOR ( 'NONE', #19070, 1000.000000000000114 ) ;
#30134=VECTOR ( 'NONE', #19190, 1000.000000000000114 ) ;
#30136=VERTEX_POINT ( 'NONE', #11011 ) ;
#30159=DIRECTION ( 'NONE',  ( 0.5200609990133008287, 0.8541291221503266584, -0.000000000000000000 ) ) ;
#30168=CARTESIAN_POINT ( 'NONE',  ( -11.59517495878806947, -96.12423995607481686, -5.500000000000000000 ) ) ;
#30172=PLANE ( 'NONE',  #6473 ) ;
#30174=DIRECTION ( 'NONE',  ( -0.1276937514489705217, -0.9918136447140101231, 0.000000000000000000 ) ) ;
#30177=VECTOR ( 'NONE', #5908, 1000.000000000000227 ) ;
#30197=CLOSED_SHELL ( 'NONE', ( #23773, #19382, #31211, #18844, #48344, #41660, #1087, #18705, #38348, #17613, #40770, #6634, #4563, #30593, #28834, #8414, #3838, #3090, #34024, #25034, #1887, #38652, #43912, #48017, #37405, #16948, #37397, #30235, #43539, #385, #46806, #27210, #16816, #28515, #16463, #7281, #24707, #19877, #3323, #34522, #41732, #34360, #40401, #20400, #20548, #11709, #4243, #36635, #8058, #31756, #25239, #33421, #21232, #22589, #36288, #10957, #4085, #41669, #44739, #3544, #48405, #23464, #25175, #32917, #13092, #22315, #4765, #33650, #16436, #29066, #5666, #27244, #30676, #38360, #5314, #1517, #29553, #47727, #2834, #35089, #38089, #34181, #15526, #33854, #46650, #47264, #41798, #17602, #10215, #29171, #38316, #41486, #36350, #19103, #29980, #43327, #17897, #5814, #43104, #1949, #3616, #36898, #46155, #44982, #25465, #1712, #17213, #43722, #14296, #7405, #3524, #35425, #43168, #20446, #3981, #16458, #41196, #12633, #10631, #6077, #12954, #37259, #21980, #45212, #46022, #23648, #30523, #20769, #47991, #21376, #7061, #46463, #2372, #28015, #22268, #1103, #40037, #9862, #44834, #32869, #40125, #1339, #33472, #41336, #5878, #39982, #5473, #21064, #20320, #45206, #46671, #14879, #14818, #16619, #11415, #29118, #14377, #16037, #30561, #47768, #36266, #6849, #31344, #20051, #3354, #29785, #17840, #25143, #33680, #27246 ) ) ;
#30200=EDGE_LOOP ( 'NONE', ( #40577, #23019, #26015, #33600 ) ) ;
#30217=ORIENTED_EDGE ( 'NONE', *, *, #39969, .F. ) ;
#30221=CARTESIAN_POINT ( 'NONE',  ( 0.000000000000000000, -120.0000000000000000, -5.500000000000000000 ) ) ;
#30230=CARTESIAN_POINT ( 'NONE',  ( -16.06301359042743115, -102.7814171781257357, -5.500000000000000000 ) ) ;
#30235=ADVANCED_FACE ( 'NONE', ( #11507 ), #26186, .F. ) ;
#30240=VERTEX_POINT ( 'NONE', #1207 ) ;
#30252=CARTESIAN_POINT ( 'NONE',  ( -21.67772167707813935, -110.8034581014852762, 5.500000000000000000 ) ) ;
#30261=EDGE_CURVE ( 'NONE', #17177, #2793, #38406, .T. ) ;
#30269=ORIENTED_EDGE ( 'NONE', *, *, #16103, .F. ) ;
#30272=FACE_OUTER_BOUND ( 'NONE', #21817, .T. ) ;
#30298=DIRECTION ( 'NONE',  ( -0.4279312458752990711, -0.9038112904824846527, 0.000000000000000000 ) ) ;
#30304=EDGE_CURVE ( 'NONE', #10011, #30136, #1453, .T. ) ;
#30311=CARTESIAN_POINT ( 'NONE',  ( -23.30023580412278505, -123.4057321492263384, 2.500000000000000000 ) ) ;
#30322=DIRECTION ( 'NONE',  ( -0.02332147558787823344, -0.9997280174009349762, 0.000000000000000000 ) ) ;
#30336=CARTESIAN_POINT ( 'NONE',  ( 16.30584220631899228, -140.9432449716519784, 5.500000000000000000 ) ) ;
#30353=DIRECTION ( 'NONE',  ( -0.08130631524010117905, 0.9966891607226784355, 0.000000000000000000 ) ) ;
#30360=DIRECTION ( 'NONE',  ( -0.000000000000000000, -0.000000000000000000, -1.000000000000000000 ) ) ;
#30371=EDGE_LOOP ( 'NONE', ( #8994, #7297, #12561, #29626 ) ) ;
#30396=PLANE ( 'NONE',  #1206 ) ;
#30406=DIRECTION ( 'NONE',  ( 0.9827303690289279636, 0.1850432970638682395, -0.000000000000000000 ) ) ;
#30419=EDGE_LOOP ( 'NONE', ( #42847, #14669, #10926, #46237 ) ) ;
#30427=DIRECTION ( 'NONE',  ( 0.4796670183876317051, -0.8774505977381971134, 0.000000000000000000 ) ) ;
#30435=DIRECTION ( 'NONE',  ( 0.8541291221503265474, -0.5200609990133007177, 0.000000000000000000 ) ) ;
#30446=VERTEX_POINT ( 'NONE', #28607 ) ;
#30463=PLANE ( 'NONE',  #17639 ) ;
#30490=CIRCLE ( 'NONE', #7039, 32.50000000000000000 ) ;
#30503=CARTESIAN_POINT ( 'NONE',  ( 19.29194287201271862, -133.5026271600380880, 2.500000000000000000 ) ) ;
#30511=FACE_OUTER_BOUND ( 'NONE', #47157, .T. ) ;
#30514=CARTESIAN_POINT ( 'NONE',  ( -20.30386590532152979, -102.9045904027214959, 5.500000000000000000 ) ) ;
#30523=ADVANCED_FACE ( 'NONE', ( #22467 ), #10956, .F. ) ;
#30541=VECTOR ( 'NONE', #24651, 1000.000000000000114 ) ;
#30546=EDGE_CURVE ( 'NONE', #17177, #30774, #14150, .T. ) ;
#30549=AXIS2_PLACEMENT_3D ( 'NONE', #37648, #29577, #37406 ) ;
#30558=DIRECTION ( 'NONE',  ( 0.3853207896976533209, -0.9227826878668545785, 0.000000000000000000 ) ) ;
#30561=ADVANCED_FACE ( 'NONE', ( #44724 ), #36650, .F. ) ;
#30570=DIRECTION ( 'NONE',  ( -0.2306669878475648139, -0.9730327541852491491, 0.000000000000000000 ) ) ;
#30575=DIRECTION ( 'NONE',  ( -0.7273375899149793211, 0.6862798483830554463, 0.000000000000000000 ) ) ;
#30577=PLANE ( 'NONE',  #42848 ) ;
#30593=ADVANCED_FACE ( 'NONE', ( #41309 ), #32979, .F. ) ;
#30595=VECTOR ( 'NONE', #13455, 1000.000000000000114 ) ;
#30604=ORIENTED_EDGE ( 'NONE', *, *, #22151, .T. ) ;
#30618=VECTOR ( 'NONE', #32650, 1000.000000000000114 ) ;
#30619=LINE ( 'NONE', #41891, #1391 ) ;
#30621=VERTEX_POINT ( 'NONE', #3111 ) ;
#30623=DIRECTION ( 'NONE',  ( -0.000000000000000000, -0.000000000000000000, -1.000000000000000000 ) ) ;
#30640=VECTOR ( 'NONE', #31291, 1000.000000000000000 ) ;
#30643=CARTESIAN_POINT ( 'NONE',  ( 16.30584220631899228, -140.9432449716519784, 2.500000000000000000 ) ) ;
#30655=EDGE_CURVE ( 'NONE', #27838, #16956, #37627, .T. ) ;
#30659=FACE_OUTER_BOUND ( 'NONE', #29507, .T. ) ;
#30676=ADVANCED_FACE ( 'NONE', ( #5486 ), #8654, .F. ) ;
#30685=CARTESIAN_POINT ( 'NONE',  ( 23.11608002360578240, -124.4885236261218182, 5.500000000000000000 ) ) ;
#30716=VECTOR ( 'NONE', #25758, 1000.000000000000227 ) ;
#30718=EDGE_CURVE ( 'NONE', #35674, #45129, #20167, .T. ) ;
#30728=ORIENTED_EDGE ( 'NONE', *, *, #36951, .T. ) ;
#30742=PLANE ( 'NONE',  #42764 ) ;
#30747=DIRECTION ( 'NONE',  ( -0.1850432970638656582, 0.9827303690289285187, 0.000000000000000000 ) ) ;
#30749=CARTESIAN_POINT ( 'NONE',  ( -15.44521549751111422, -137.7748507232956001, 5.500000000000000000 ) ) ;
#30760=LINE ( 'NONE', #4092, #33714 ) ;
#30774=VERTEX_POINT ( 'NONE', #34853 ) ;
#30792=EDGE_CURVE ( 'NONE', #38227, #39318, #39988, .T. ) ;
#30794=AXIS2_PLACEMENT_3D ( 'NONE', #18766, #29073, #41078 ) ;
#30801=DIRECTION ( 'NONE',  ( -0.5200609990132993854, -0.8541291221503274356, 0.000000000000000000 ) ) ;
#30819=VERTEX_POINT ( 'NONE', #10612 ) ;
#30824=PLANE ( 'NONE',  #34762 ) ;
#30826=CARTESIAN_POINT ( 'NONE',  ( -16.07206065793331007, -141.0698568150738197, -2.500000000000000000 ) ) ;
#30829=CARTESIAN_POINT ( 'NONE',  ( 0.000000000000000000, -120.0000000000000000, 2.500000000000000000 ) ) ;
#30848=EDGE_CURVE ( 'NONE', #28620, #35445, #9622, .T. ) ;
#30851=ORIENTED_EDGE ( 'NONE', *, *, #22151, .F. ) ;
#30858=LINE ( 'NONE', #45788, #23524 ) ;
#30859=ORIENTED_EDGE ( 'NONE', *, *, #17001, .F. ) ;
#30865=ORIENTED_EDGE ( 'NONE', *, *, #17969, .F. ) ;
#30870=ORIENTED_EDGE ( 'NONE', *, *, #22373, .T. ) ;
#30879=CARTESIAN_POINT ( 'NONE',  ( -14.87942725330654348, -141.9795960975983178, 5.500000000000000000 ) ) ;
#30905=VERTEX_POINT ( 'NONE', #39755 ) ;
#30930=VECTOR ( 'NONE', #16296, 1000.000000000000114 ) ;
#30961=VECTOR ( 'NONE', #40838, 1000.000000000000000 ) ;
#30963=FACE_OUTER_BOUND ( 'NONE', #23752, .T. ) ;
#30964=ORIENTED_EDGE ( 'NONE', *, *, #5688, .F. ) ;
#30980=ORIENTED_EDGE ( 'NONE', *, *, #6251, .T. ) ;
#30984=DIRECTION ( 'NONE',  ( -0.3311129884571295534, -0.9435911131814398445, 0.000000000000000000 ) ) ;
#31001=DIRECTION ( 'NONE',  ( 0.9827303690289282967, 0.1850432970638667407, -0.000000000000000000 ) ) ;
#31008=DIRECTION ( 'NONE',  ( -0.1850432970638667129, 0.9827303690289281857, 0.000000000000000000 ) ) ;
#31011=EDGE_CURVE ( 'NONE', #29568, #19113, #44376, .T. ) ;
#31022=DIRECTION ( 'NONE',  ( 0.08130631524010120681, -0.9966891607226784355, 0.000000000000000000 ) ) ;
#31039=ORIENTED_EDGE ( 'NONE', *, *, #45493, .T. ) ;
#31052=CARTESIAN_POINT ( 'NONE',  ( 2.874421927457452952, -143.3717286177755739, -5.500000000000000000 ) ) ;
#31065=CARTESIAN_POINT ( 'NONE',  ( 12.50000000000000000, -132.5000000000000000, 2.500000000000000000 ) ) ;
#31078=DIRECTION ( 'NONE',  ( -0.9997280174009349762, 0.02332147558787671729, 0.000000000000000000 ) ) ;
#31082=ORIENTED_EDGE ( 'NONE', *, *, #3472, .F. ) ;
#31095=AXIS2_PLACEMENT_3D ( 'NONE', #4096, #164, #31022 ) ;
#31106=DIRECTION ( 'NONE',  ( -1.000000000000000000, 0.000000000000000000, 0.000000000000000000 ) ) ;
#31109=ORIENTED_EDGE ( 'NONE', *, *, #11664, .T. ) ;
#31112=AXIS2_PLACEMENT_3D ( 'NONE', #1113, #31001, #23625 ) ;
#31118=ORIENTED_EDGE ( 'NONE', *, *, #40004, .T. ) ;
#31124=PLANE ( 'NONE',  #3392 ) ;
#31125=CARTESIAN_POINT ( 'NONE',  ( -3.961125083139900749, -143.2122702051246677, 5.500000000000000000 ) ) ;
#31161=CARTESIAN_POINT ( 'NONE',  ( -21.67772167707813935, -110.8034581014852762, 2.500000000000000000 ) ) ;
#31163=ORIENTED_EDGE ( 'NONE', *, *, #14480, .F. ) ;
#31165=VECTOR ( 'NONE', #33219, 1000.000000000000114 ) ;
#31166=VECTOR ( 'NONE', #41038, 1000.000000000000114 ) ;
#31186=FACE_OUTER_BOUND ( 'NONE', #39315, .T. ) ;
#31211=ADVANCED_FACE ( 'NONE', ( #40411 ), #17151, .T. ) ;
#31216=DIRECTION ( 'NONE',  ( 0.02332147558787931590, 0.9997280174009348652, -0.000000000000000000 ) ) ;
#31233=LINE ( 'NONE', #1605, #30930 ) ;
#31237=CARTESIAN_POINT ( 'NONE',  ( 23.49916127795269460, -121.5130826919798039, 5.500000000000000000 ) ) ;
#31243=CARTESIAN_POINT ( 'NONE',  ( -0.9515373497862389396, -96.47140937769621871, 5.500000000000000000 ) ) ;
#31246=PLANE ( 'NONE',  #16840 ) ;
#31266=AXIS2_PLACEMENT_3D ( 'NONE', #27945, #43094, #20319 ) ;
#31275=VECTOR ( 'NONE', #32823, 1000.000000000000000 ) ;
#31282=LINE ( 'NONE', #24166, #3754 ) ;
#31283=DIRECTION ( 'NONE',  ( -0.9997280174009349762, 0.02332147558787671729, 0.000000000000000000 ) ) ;
#31291=DIRECTION ( 'NONE',  ( -0.000000000000000000, -0.000000000000000000, -1.000000000000000000 ) ) ;
#31323=( NAMED_UNIT ( * ) PLANE_ANGLE_UNIT ( ) SI_UNIT ( $, .RADIAN. ) );
#31328=FACE_OUTER_BOUND ( 'NONE', #17202, .T. ) ;
#31336=VECTOR ( 'NONE', #33059, 1000.000000000000000 ) ;
#31344=ADVANCED_FACE ( 'NONE', ( #41135 ), #26194, .T. ) ;
#31355=ORIENTED_EDGE ( 'NONE', *, *, #16091, .T. ) ;
#31359=DIRECTION ( 'NONE',  ( 1.000000000000000000, 0.000000000000000000, 0.000000000000000000 ) ) ;
#31386=CARTESIAN_POINT ( 'NONE',  ( 6.377742925735834234, -145.7647898336708181, 5.500000000000000000 ) ) ;
#31399=EDGE_LOOP ( 'NONE', ( #44142, #46167, #39864, #43537 ) ) ;
#31412=FACE_BOUND ( 'NONE', #32283, .T. ) ;
#31423=VERTEX_POINT ( 'NONE', #33760 ) ;
#31429=CARTESIAN_POINT ( 'NONE',  ( 0.000000000000000000, -120.0000000000000000, -2.500000000000000000 ) ) ;
#31439=CARTESIAN_POINT ( 'NONE',  ( 25.81725066941077529, -113.8380548628854854, 5.500000000000000000 ) ) ;
#31442=ORIENTED_EDGE ( 'NONE', *, *, #25767, .T. ) ;
#31449=EDGE_LOOP ( 'NONE', ( #21477, #45679, #4428, #48408 ) ) ;
#31469=AXIS2_PLACEMENT_3D ( 'NONE', #45921, #47528, #13109 ) ;
#31472=PLANE ( 'NONE',  #3679 ) ;
#31482=VECTOR ( 'NONE', #2053, 1000.000000000000114 ) ;
#31485=CARTESIAN_POINT ( 'NONE',  ( 19.29194287201271862, -133.5026271600380880, 5.500000000000000000 ) ) ;
#31486=FACE_OUTER_BOUND ( 'NONE', #39673, .T. ) ;
#31489=FACE_OUTER_BOUND ( 'NONE', #5980, .T. ) ;
#31493=DIRECTION ( 'NONE',  ( -0.6064928550163511956, -0.7950889364178798102, 0.000000000000000000 ) ) ;
#31494=LINE ( 'NONE', #30514, #37787 ) ;
#31503=ORIENTED_EDGE ( 'NONE', *, *, #41221, .T. ) ;
#31529=CARTESIAN_POINT ( 'NONE',  ( -0.1915406271734583221, -121.4877204670710427, -2.500000000000000000 ) ) ;
#31544=ORIENTED_EDGE ( 'NONE', *, *, #24767, .T. ) ;
#31547=DIRECTION ( 'NONE',  ( 0.1276937514489694392, 0.9918136447140102341, -0.000000000000000000 ) ) ;
#31566=AXIS2_PLACEMENT_3D ( 'NONE', #9167, #16990, #28252 ) ;
#31592=ORIENTED_EDGE ( 'NONE', *, *, #26203, .F. ) ;
#31612=DIRECTION ( 'NONE',  ( 0.6691306063588671194, -0.7431448254773862505, 0.000000000000000000 ) ) ;
#31621=AXIS2_PLACEMENT_3D ( 'NONE', #6194, #24793, #39968 ) ;
#31629=EDGE_CURVE ( 'NONE', #35538, #24295, #15352, .T. ) ;
#31631=ORIENTED_EDGE ( 'NONE', *, *, #28874, .F. ) ;
#31654=LINE ( 'NONE', #35291, #3546 ) ;
#31657=ORIENTED_EDGE ( 'NONE', *, *, #29733, .T. ) ;
#31674=CARTESIAN_POINT ( 'NONE',  ( 22.08297821871651934, -111.8242998470044540, 5.500000000000000000 ) ) ;
#31676=EDGE_LOOP ( 'NONE', ( #18186, #42397, #13920, #18452 ) ) ;
#31697=CIRCLE ( 'NONE', #1157, 35.50000000000000711 ) ;
#31715=PLANE ( 'NONE',  #8234 ) ;
#31716=ORIENTED_EDGE ( 'NONE', *, *, #33962, .F. ) ;
#31727=EDGE_LOOP ( 'NONE', ( #38568, #22948, #31716, #3291 ) ) ;
#31728=FACE_OUTER_BOUND ( 'NONE', #47965, .T. ) ;
#31729=VERTEX_POINT ( 'NONE', #11442 ) ;
#31731=DIRECTION ( 'NONE',  ( 0.3311129884571280546, 0.9435911131814402886, 0.000000000000000000 ) ) ;
#31735=DIRECTION ( 'NONE',  ( 0.8541291221503261033, -0.5200609990133016058, 0.000000000000000000 ) ) ;
#31739=DIRECTION ( 'NONE',  ( 0.8541291221503275466, -0.5200609990132993854, 0.000000000000000000 ) ) ;
#31748=LINE ( 'NONE', #46662, #8082 ) ;
#31756=ADVANCED_FACE ( 'NONE', ( #31486 ), #39058, .F. ) ;
#31760=VECTOR ( 'NONE', #26059, 1000.000000000000000 ) ;
#31780=CARTESIAN_POINT ( 'NONE',  ( 0.5480546763151027401, -96.50639159107802811, 2.500000000000000000 ) ) ;
#31782=EDGE_CURVE ( 'NONE', #39583, #40958, #4799, .T. ) ;
#31807=DIRECTION ( 'NONE',  ( -0.000000000000000000, -0.000000000000000000, -1.000000000000000000 ) ) ;
#31828=ORIENTED_EDGE ( 'NONE', *, *, #20504, .T. ) ;
#31838=VERTEX_POINT ( 'NONE', #1861 ) ;
#31839=CARTESIAN_POINT ( 'NONE',  ( -20.30386590532152979, -102.9045904027214959, 2.500000000000000000 ) ) ;
#31847=ORIENTED_EDGE ( 'NONE', *, *, #40242, .F. ) ;
#31851=LINE ( 'NONE', #32722, #15494 ) ;
#31860=CARTESIAN_POINT ( 'NONE',  ( -5.420674214417706693, -142.8662697233533265, 2.500000000000000000 ) ) ;
#31872=LINE ( 'NONE', #43353, #31940 ) ;
#31900=ORIENTED_EDGE ( 'NONE', *, *, #7698, .F. ) ;
#31909=ORIENTED_EDGE ( 'NONE', *, *, #27715, .T. ) ;
#31912=AXIS2_PLACEMENT_3D ( 'NONE', #18422, #30174, #544 ) ;
#31935=DIRECTION ( 'NONE',  ( 0.9966891607226785466, 0.08130631524009969413, -0.000000000000000000 ) ) ;
#31940=VECTOR ( 'NONE', #39915, 1000.000000000000000 ) ;
#31973=DIRECTION ( 'NONE',  ( -0.1276937514489679404, -0.9918136447140103451, 0.000000000000000000 ) ) ;
#31985=EDGE_CURVE ( 'NONE', #28510, #42762, #43208, .T. ) ;
#31990=DIRECTION ( 'NONE',  ( 0.000000000000000000, 0.000000000000000000, 1.000000000000000000 ) ) ;
#32015=CARTESIAN_POINT ( 'NONE',  ( 4.903647372192503795, -146.0423547792665886, -2.500000000000000000 ) ) ;
#32017=LINE ( 'NONE', #12439, #30640 ) ;
#32026=DIRECTION ( 'NONE',  ( -0.5687579148473743684, 0.8225049752423791993, 0.000000000000000000 ) ) ;
#32046=ORIENTED_EDGE ( 'NONE', *, *, #17001, .T. ) ;
#32049=VERTEX_POINT ( 'NONE', #40548 ) ;
#32051=PLANE ( 'NONE',  #35528 ) ;
#32069=CARTESIAN_POINT ( 'NONE',  ( 0.1219594728601484379, -121.4950337410840149, -2.500000000000000000 ) ) ;
#32074=ORIENTED_EDGE ( 'NONE', *, *, #41122, .T. ) ;
#32086=CARTESIAN_POINT ( 'NONE',  ( -35.50000000000000711, -120.0000000000000000, 2.500000000000000000 ) ) ;
#32087=PLANE ( 'NONE',  #43720 ) ;
#32088=CARTESIAN_POINT ( 'NONE',  ( 12.13205353604972991, -140.1820037904669789, 2.500000000000000000 ) ) ;
#32089=EDGE_CURVE ( 'NONE', #21999, #41940, #11654, .T. ) ;
#32090=LINE ( 'NONE', #16911, #30177 ) ;
#32104=DIRECTION ( 'NONE',  ( 1.000000000000000000, 0.000000000000000000, 0.000000000000000000 ) ) ;
#32115=ORIENTED_EDGE ( 'NONE', *, *, #10889, .T. ) ;
#32123=ORIENTED_EDGE ( 'NONE', *, *, #32656, .T. ) ;
#32127=FACE_BOUND ( 'NONE', #35236, .T. ) ;
#32168=VERTEX_POINT ( 'NONE', #3581 ) ;
#32180=CARTESIAN_POINT ( 'NONE',  ( 5.822613034544236399, -142.8165987265839476, -2.500000000000000000 ) ) ;
#32187=LINE ( 'NONE', #47571, #6977 ) ;
#32188=CARTESIAN_POINT ( 'NONE',  ( 3.429551818649054340, -146.3199197248623875, -2.500000000000000444 ) ) ;
#32214=EDGE_CURVE ( 'NONE', #30774, #47208, #31233, .T. ) ;
#32215=CARTESIAN_POINT ( 'NONE',  ( -17.26469406256017791, -140.1601175325492648, 5.500000000000000000 ) ) ;
#32225=EDGE_LOOP ( 'NONE', ( #27055, #22794, #21620, #24908 ) ) ;
#32246=CARTESIAN_POINT ( 'NONE',  ( 114.1267819554180392, -82.91796067500511924, -5.500000000000000000 ) ) ;
#32251=FACE_BOUND ( 'NONE', #47785, .T. ) ;
#32253=CARTESIAN_POINT ( 'NONE',  ( -21.33958957442910886, -129.9559990355020034, 5.500000000000000000 ) ) ;
#32264=LINE ( 'NONE', #35698, #21019 ) ;
#32267=ORIENTED_EDGE ( 'NONE', *, *, #8962, .F. ) ;
#32277=ORIENTED_EDGE ( 'NONE', *, *, #42893, .F. ) ;
#32283=EDGE_LOOP ( 'NONE', ( #15449, #48353, #18159, #29042 ) ) ;
#32295=EDGE_LOOP ( 'NONE', ( #29424, #41568, #45450, #2170 ) ) ;
#32304=ORIENTED_EDGE ( 'NONE', *, *, #30655, .F. ) ;
#32330=FACE_OUTER_BOUND ( 'NONE', #22768, .T. ) ;
#32351=VECTOR ( 'NONE', #6872, 1000.000000000000000 ) ;
#32356=EDGE_CURVE ( 'NONE', #9579, #36733, #28520, .T. ) ;
#32359=DIRECTION ( 'NONE',  ( 0.9135454576426004225, 0.4067366430758009854, 0.000000000000000000 ) ) ;
#32364=DIRECTION ( 'NONE',  ( -0.8774505977381983346, -0.4796670183876294291, 0.000000000000000000 ) ) ;
#32383=CARTESIAN_POINT ( 'NONE',  ( -22.53294031248082163, -134.0273518838794757, 5.500000000000000000 ) ) ;
#32387=CARTESIAN_POINT ( 'NONE',  ( 20.10151712711562766, -102.7321394148470830, 2.500000000000000000 ) ) ;
#32400=EDGE_LOOP ( 'NONE', ( #32792, #46044, #7446, #9746 ) ) ;
#32420=CARTESIAN_POINT ( 'NONE',  ( 5.822613034544236399, -142.8165987265839760, -5.500000000000000000 ) ) ;
#32421=DIRECTION ( 'NONE',  ( 0.6516173805718078471, -0.7585478161175706058, 0.000000000000000000 ) ) ;
#32431=CARTESIAN_POINT ( 'NONE',  ( 0.000000000000000000, -89.50000000000000000, 5.500000000000000000 ) ) ;
#32433=ORIENTED_EDGE ( 'NONE', *, *, #34114, .T. ) ;
#32453=FACE_OUTER_BOUND ( 'NONE', #38638, .T. ) ;
#32462=EDGE_CURVE ( 'NONE', #15896, #35257, #18200, .T. ) ;
#32478=DIRECTION ( 'NONE',  ( -0.3853207896976523772, 0.9227826878668550226, 0.000000000000000000 ) ) ;
#32490=DIRECTION ( 'NONE',  ( 1.000000000000000000, 0.000000000000000000, -0.000000000000000000 ) ) ;
#32496=FILL_AREA_STYLE ('',( #21470 ) ) ;
#32498=ORIENTED_EDGE ( 'NONE', *, *, #21260, .F. ) ;
#32500=ORIENTED_EDGE ( 'NONE', *, *, #8189, .T. ) ;
#32548=VECTOR ( 'NONE', #30801, 1000.000000000000000 ) ;
#32553=ORIENTED_EDGE ( 'NONE', *, *, #10263, .F. ) ;
#32577=APPLICATION_CONTEXT ( 'automotive_design' ) ;
#32594=PLANE ( 'NONE',  #34093 ) ;
#32597=VERTEX_POINT ( 'NONE', #38506 ) ;
#32627=ORIENTED_EDGE ( 'NONE', *, *, #14550, .T. ) ;
#32647=EDGE_CURVE ( 'NONE', #44807, #28358, #37779, .T. ) ;
#32650=DIRECTION ( 'NONE',  ( -0.1276937514489679404, -0.9918136447140103451, 0.000000000000000000 ) ) ;
#32656=EDGE_CURVE ( 'NONE', #8515, #1874, #24543, .T. ) ;
#32666=VECTOR ( 'NONE', #26435, 1000.000000000000000 ) ;
#32677=CARTESIAN_POINT ( 'NONE',  ( -19.27444613274700913, -101.8135840178490668, -2.500000000000000000 ) ) ;
#32679=ORIENTED_EDGE ( 'NONE', *, *, #41673, .F. ) ;
#32681=VECTOR ( 'NONE', #5913, 999.9999999999998863 ) ;
#32688=EDGE_LOOP ( 'NONE', ( #46711, #39200, #14724, #14558 ) ) ;
#32700=ORIENTED_EDGE ( 'NONE', *, *, #24660, .F. ) ;
#32721=VECTOR ( 'NONE', #2789, 1000.000000000000114 ) ;
#32722=CARTESIAN_POINT ( 'NONE',  ( -19.90058851926621131, -132.5883508287165853, 5.500000000000000000 ) ) ;
#32730=DIRECTION ( 'NONE',  ( 1.000000000000000000, 0.000000000000000000, 0.000000000000000000 ) ) ;
#32745=CARTESIAN_POINT ( 'NONE',  ( -8.826826895187510402, -94.96827758698185562, -5.500000000000000000 ) ) ;
#32757=ORIENTED_EDGE ( 'NONE', *, *, #9703, .F. ) ;
#32768=ORIENTED_EDGE ( 'NONE', *, *, #47188, .T. ) ;
#32776=DIRECTION ( 'NONE',  ( -0.6516173805718067369, 0.7585478161175716050, 0.000000000000000000 ) ) ;
#32786=DIRECTION ( 'NONE',  ( 0.9227826878668540234, 0.3853207896976547087, 0.000000000000000000 ) ) ;
#32792=ORIENTED_EDGE ( 'NONE', *, *, #9770, .T. ) ;
#32800=AXIS2_PLACEMENT_3D ( 'NONE', #35836, #2301, #17218 ) ;
#32819=ORIENTED_EDGE ( 'NONE', *, *, #6299, .F. ) ;
#32821=CARTESIAN_POINT ( 'NONE',  ( 0.000000000000000000, -120.0000000000000000, -2.500000000000000000 ) ) ;
#32823=DIRECTION ( 'NONE',  ( -0.000000000000000000, -0.000000000000000000, -1.000000000000000000 ) ) ;
#32826=ORIENTED_EDGE ( 'NONE', *, *, #36080, .T. ) ;
#32829=ORIENTED_EDGE ( 'NONE', *, *, #13169, .T. ) ;
#32830=FACE_OUTER_BOUND ( 'NONE', #9256, .T. ) ;
#32832=ORIENTED_EDGE ( 'NONE', *, *, #15862, .T. ) ;
#32847=AXIS2_PLACEMENT_3D ( 'NONE', #26944, #8327, #40900 ) ;
#32869=ADVANCED_FACE ( 'NONE', ( #48259 ), #29894, .F. ) ;
#32899=CARTESIAN_POINT ( 'NONE',  ( -15.44521549751111422, -137.7748507232956001, 5.500000000000000000 ) ) ;
#32903=ORIENTED_EDGE ( 'NONE', *, *, #16929, .T. ) ;
#32917=ADVANCED_FACE ( 'NONE', ( #33794 ), #41175, .F. ) ;
#32941=DIRECTION ( 'NONE',  ( 0.6064928550163524168, 0.7950889364178788110, -0.000000000000000000 ) ) ;
#32943=CIRCLE ( 'NONE', #22008, 32.50000000000000000 ) ;
#32967=AXIS2_PLACEMENT_3D ( 'NONE', #29349, #21985, #36445 ) ;
#32970=CARTESIAN_POINT ( 'NONE',  ( 0.000000000000000000, -120.0000000000000000, 2.500000000000000000 ) ) ;
#32976=CARTESIAN_POINT ( 'NONE',  ( -119.3426274441927433, -132.5434155921188619, 5.500000000000000000 ) ) ;
#32979=PLANE ( 'NONE',  #38515 ) ;
#32986=EDGE_CURVE ( 'NONE', #13936, #5271, #15460, .T. ) ;
#32993=FACE_OUTER_BOUND ( 'NONE', #30371, .T. ) ;
#32995=ORIENTED_EDGE ( 'NONE', *, *, #8553, .T. ) ;
#33018=FACE_OUTER_BOUND ( 'NONE', #37717, .T. ) ;
#33022=CARTESIAN_POINT ( 'NONE',  ( -23.97194136764370498, -131.3950000906648938, 5.500000000000000000 ) ) ;
#33023=AXIS2_PLACEMENT_3D ( 'NONE', #30221, #19905, #15293 ) ;
#33032=CARTESIAN_POINT ( 'NONE',  ( -22.17439115976385366, -112.2188447712574799, 2.500000000000000000 ) ) ;
#33046=CARTESIAN_POINT ( 'NONE',  ( -30.50000000000000000, -120.0000000000000000, 2.500000000000000000 ) ) ;
#33049=VECTOR ( 'NONE', #5644, 1000.000000000000000 ) ;
#33059=DIRECTION ( 'NONE',  ( -0.000000000000000000, -0.000000000000000000, -1.000000000000000000 ) ) ;
#33067=EDGE_LOOP ( 'NONE', ( #9296, #15747, #44927, #11886 ) ) ;
#33082=FACE_OUTER_BOUND ( 'NONE', #23254, .T. ) ;
#33083=VERTEX_POINT ( 'NONE', #42855 ) ;
#33099=DIRECTION ( 'NONE',  ( -0.000000000000000000, -0.000000000000000000, -1.000000000000000000 ) ) ;
#33108=VECTOR ( 'NONE', #22030, 1000.000000000000000 ) ;
#33116=VECTOR ( 'NONE', #4416, 1000.000000000000114 ) ;
#33167=DIRECTION ( 'NONE',  ( 0.6064928550163524168, 0.7950889364178788110, -0.000000000000000000 ) ) ;
#33173=VECTOR ( 'NONE', #11082, 1000.000000000000114 ) ;
#33185=ORIENTED_EDGE ( 'NONE', *, *, #29185, .T. ) ;
#33189=VERTEX_POINT ( 'NONE', #46775 ) ;
#33195=LINE ( 'NONE', #6773, #11590 ) ;
#33208=CARTESIAN_POINT ( 'NONE',  ( -18.12185313557660038, -104.9634299478706794, 5.500000000000000000 ) ) ;
#33219=DIRECTION ( 'NONE',  ( 0.9997280174009349762, -0.02332147558787674158, 0.000000000000000000 ) ) ;
#33223=CARTESIAN_POINT ( 'NONE',  ( 24.95699195200416654, -110.9640411295978595, -5.500000000000000000 ) ) ;
#33245=DIRECTION ( 'NONE',  ( -0.9227826878668540234, -0.3853207896976547642, 0.000000000000000000 ) ) ;
#33265=VECTOR ( 'NONE', #38957, 1000.000000000000000 ) ;
#33309=PLANE ( 'NONE',  #32847 ) ;
#33323=FACE_BOUND ( 'NONE', #15353, .T. ) ;
#33326=CARTESIAN_POINT ( 'NONE',  ( 2.874421927457452952, -143.3717286177755739, 5.500000000000000000 ) ) ;
#33336=FACE_OUTER_BOUND ( 'NONE', #47789, .T. ) ;
#33337=CARTESIAN_POINT ( 'NONE',  ( -14.25258209288423750, -138.6845900058201551, -2.500000000000000000 ) ) ;
#33340=LINE ( 'NONE', #14743, #17155 ) ;
#33349=CARTESIAN_POINT ( 'NONE',  ( 14.59956846177685996, -138.4757300459248484, -2.500000000000000000 ) ) ;
#33372=PLANE ( 'NONE',  #8598 ) ;
#33374=EDGE_LOOP ( 'NONE', ( #4141, #5097, #28459, #34710 ) ) ;
#33378=EDGE_CURVE ( 'NONE', #47615, #14593, #15821, .T. ) ;
#33393=LINE ( 'NONE', #44645, #27501 ) ;
#33396=DIRECTION ( 'NONE',  ( 0.1276937514489679404, 0.9918136447140103451, 0.000000000000000000 ) ) ;
#33398=DIRECTION ( 'NONE',  ( 0.9580045777625458836, 0.2867529058022011412, -0.000000000000000000 ) ) ;
#33407=CARTESIAN_POINT ( 'NONE',  ( -17.26469406256017791, -140.1601175325492648, -2.500000000000000444 ) ) ;
#33409=VECTOR ( 'NONE', #11138, 1000.000000000000114 ) ;
#33414=DIRECTION ( 'NONE',  ( -0.000000000000000000, -0.000000000000000000, -1.000000000000000000 ) ) ;
#33421=ADVANCED_FACE ( 'NONE', ( #31489 ), #9199, .F. ) ;
#33426=VECTOR ( 'NONE', #8251, 1000.000000000000000 ) ;
#33429=PLANE ( 'NONE',  #28499 ) ;
#33446=CARTESIAN_POINT ( 'NONE',  ( -24.94940289813038703, -237.3777120880567963, 5.500000000000000000 ) ) ;
#33456=VECTOR ( 'NONE', #18987, 1000.000000000000227 ) ;
#33467=DIRECTION ( 'NONE',  ( -0.000000000000000000, -0.000000000000000000, -1.000000000000000000 ) ) ;
#33472=ADVANCED_FACE ( 'NONE', ( #16307 ), #31246, .F. ) ;
#33473=ORIENTED_EDGE ( 'NONE', *, *, #44642, .F. ) ;
#33495=ORIENTED_EDGE ( 'NONE', *, *, #34557, .F. ) ;
#33504=ORIENTED_EDGE ( 'NONE', *, *, #15539, .T. ) ;
#33508=PLANE ( 'NONE',  #3429 ) ;
#33510=DIRECTION ( 'NONE',  ( 0.1276937514489679404, 0.9918136447140103451, -0.000000000000000000 ) ) ;
#33519=CIRCLE ( 'NONE', #43697, 32.50000000000000000 ) ;
#33527=DIRECTION ( 'NONE',  ( -0.000000000000000000, -0.000000000000000000, 1.000000000000000000 ) ) ;
#33578=LINE ( 'NONE', #4217, #13103 ) ;
#33600=ORIENTED_EDGE ( 'NONE', *, *, #3472, .T. ) ;
#33618=CARTESIAN_POINT ( 'NONE',  ( -21.67772167707813935, -110.8034581014852762, 5.500000000000000000 ) ) ;
#33631=CARTESIAN_POINT ( 'NONE',  ( -20.30386590532155111, -102.9045904027214959, -2.500000000000000000 ) ) ;
#33645=VECTOR ( 'NONE', #41468, 1000.000000000000114 ) ;
#33648=AXIS2_PLACEMENT_3D ( 'NONE', #14250, #40208, #29166 ) ;
#33650=ADVANCED_FACE ( 'NONE', ( #48322 ), #45143, .F. ) ;
#33668=EDGE_LOOP ( 'NONE', ( #19406, #11894, #2897, #46922 ) ) ;
#33675=DIRECTION ( 'NONE',  ( 0.7950889364178798102, -0.6064928550163511956, 0.000000000000000000 ) ) ;
#33679=EDGE_LOOP ( 'NONE', ( #47500, #33888, #35838, #24128 ) ) ;
#33680=ADVANCED_FACE ( 'NONE', ( #37065 ), #26049, .F. ) ;
#33686=EDGE_CURVE ( 'NONE', #35257, #2423, #14800, .T. ) ;
#33705=EDGE_CURVE ( 'NONE', #20259, #24269, #15043, .T. ) ;
#33714=VECTOR ( 'NONE', #26366, 1000.000000000000227 ) ;
#33727=CARTESIAN_POINT ( 'NONE',  ( 0.000000000000000000, -120.0000000000000000, 2.500000000000000000 ) ) ;
#33738=VERTEX_POINT ( 'NONE', #41238 ) ;
#33747=LINE ( 'NONE', #41121, #45105 ) ;
#33752=VECTOR ( 'NONE', #25959, 1000.000000000000114 ) ;
#33760=CARTESIAN_POINT ( 'NONE',  ( -21.33958957442910886, -129.9559990355020034, -5.500000000000000000 ) ) ;
#33783=VECTOR ( 'NONE', #44294, 1000.000000000000114 ) ;
#33787=ORIENTED_EDGE ( 'NONE', *, *, #35037, .F. ) ;
#33788=CARTESIAN_POINT ( 'NONE',  ( -12.50000000000000000, -107.5000000000000000, 2.500000000000000000 ) ) ;
#33794=FACE_OUTER_BOUND ( 'NONE', #48413, .T. ) ;
#33796=VECTOR ( 'NONE', #7475, 1000.000000000000000 ) ;
#33800=PLANE ( 'NONE',  #12825 ) ;
#33808=DIRECTION ( 'NONE',  ( -0.8225049752423776450, -0.5687579148473765889, 0.000000000000000000 ) ) ;
#33819=EDGE_CURVE ( 'NONE', #11732, #21639, #34855, .T. ) ;
#33842=ORIENTED_EDGE ( 'NONE', *, *, #16923, .T. ) ;
#33843=ORIENTED_EDGE ( 'NONE', *, *, #27471, .T. ) ;
#33850=ORIENTED_EDGE ( 'NONE', *, *, #5209, .F. ) ;
#33851=PLANE ( 'NONE',  #43553 ) ;
#33854=ADVANCED_FACE ( 'NONE', ( #5241 ), #4511, .F. ) ;
#33862=ORIENTED_EDGE ( 'NONE', *, *, #22597, .F. ) ;
#33867=LINE ( 'NONE', #36814, #2403 ) ;
#33869=DIRECTION ( 'NONE',  ( -0.000000000000000000, -0.000000000000000000, -1.000000000000000000 ) ) ;
#33871=DIRECTION ( 'NONE',  ( -0.4796670183876317051, 0.8774505977381972244, 0.000000000000000000 ) ) ;
#33887=AXIS2_PLACEMENT_3D ( 'NONE', #41128, #26433, #19071 ) ;
#33888=ORIENTED_EDGE ( 'NONE', *, *, #35651, .F. ) ;
#33907=CARTESIAN_POINT ( 'NONE',  ( 22.63442173698368620, -133.7816164738524378, 2.500000000000000000 ) ) ;
#33936=LINE ( 'NONE', #11920, #8406 ) ;
#33962=EDGE_CURVE ( 'NONE', #10970, #21061, #16906, .T. ) ;
#33973=CARTESIAN_POINT ( 'NONE',  ( 1.499592026101426168, -120.0349822133818094, 2.500000000000000000 ) ) ;
#33977=EDGE_CURVE ( 'NONE', #11749, #4261, #5712, .T. ) ;
#33980=ORIENTED_EDGE ( 'NONE', *, *, #17112, .F. ) ;
#33984=CARTESIAN_POINT ( 'NONE',  ( -7.670864526094549163, -97.73662565058241114, 5.500000000000000000 ) ) ;
#33987=VERTEX_POINT ( 'NONE', #14014 ) ;
#34002=CARTESIAN_POINT ( 'NONE',  ( 22.08297821871651934, -111.8242998470044540, -5.500000000000000000 ) ) ;
#34024=ADVANCED_FACE ( 'NONE', ( #6679 ), #24555, .F. ) ;
#34025=VECTOR ( 'NONE', #33871, 999.9999999999998863 ) ;
#34033=ORIENTED_EDGE ( 'NONE', *, *, #7782, .F. ) ;
#34042=VERTEX_POINT ( 'NONE', #5970 ) ;
#34062=LINE ( 'NONE', #25746, #45518 ) ;
#34074=PLANE ( 'NONE',  #2590 ) ;
#34082=ORIENTED_EDGE ( 'NONE', *, *, #18561, .F. ) ;
#34091=ORIENTED_EDGE ( 'NONE', *, *, #7698, .T. ) ;
#34093=AXIS2_PLACEMENT_3D ( 'NONE', #13994, #28913, #43847 ) ;
#34107=DIRECTION ( 'NONE',  ( 0.9827303690289279636, 0.1850432970638681840, 0.000000000000000000 ) ) ;
#34114=EDGE_CURVE ( 'NONE', #5335, #29594, #47767, .T. ) ;
#34132=ORIENTED_EDGE ( 'NONE', *, *, #35711, .T. ) ;
#34144=CARTESIAN_POINT ( 'NONE',  ( 2.047646702416564768, -96.54137380445985173, -5.500000000000000000 ) ) ;
#34146=EDGE_CURVE ( 'NONE', #6148, #19113, #7637, .T. ) ;
#34164=DIRECTION ( 'NONE',  ( -1.000000000000000000, 0.000000000000000000, 0.000000000000000000 ) ) ;
#34166=FACE_OUTER_BOUND ( 'NONE', #17955, .T. ) ;
#34181=ADVANCED_FACE ( 'NONE', ( #48266 ), #4213, .F. ) ;
#34199=VERTEX_POINT ( 'NONE', #11067 ) ;
#34212=ORIENTED_EDGE ( 'NONE', *, *, #46, .T. ) ;
#34213=ORIENTED_EDGE ( 'NONE', *, *, #42992, .T. ) ;
#34219=ORIENTED_EDGE ( 'NONE', *, *, #18778, .F. ) ;
#34220=ORIENTED_EDGE ( 'NONE', *, *, #21305, .T. ) ;
#34222=FACE_OUTER_BOUND ( 'NONE', #5332, .T. ) ;
#34232=CARTESIAN_POINT ( 'NONE',  ( 23.30762065077924916, -123.0008031590507329, -2.500000000000000000 ) ) ;
#34239=PLANE ( 'NONE',  #42628 ) ;
#34240=FACE_OUTER_BOUND ( 'NONE', #48404, .T. ) ;
#34251=ORIENTED_EDGE ( 'NONE', *, *, #42609, .T. ) ;
#34252=EDGE_CURVE ( 'NONE', #27123, #26989, #26723, .T. ) ;
#34261=ORIENTED_EDGE ( 'NONE', *, *, #32462, .T. ) ;
#34272=DIRECTION ( 'NONE',  ( -0.000000000000000000, -0.000000000000000000, 1.000000000000000000 ) ) ;
#34280=ORIENTED_EDGE ( 'NONE', *, *, #28083, .F. ) ;
#34307=CARTESIAN_POINT ( 'NONE',  ( 22.94323693612312809, -114.6983135802921083, 5.500000000000000000 ) ) ;
#34333=DIRECTION ( 'NONE',  ( -0.000000000000000000, -0.000000000000000000, -1.000000000000000000 ) ) ;
#34357=EDGE_LOOP ( 'NONE', ( #32304, #44213, #44454, #4534 ) ) ;
#34360=ADVANCED_FACE ( 'NONE', ( #17140 ), #16910, .F. ) ;
#34363=VERTEX_POINT ( 'NONE', #32088 ) ;
#34365=CARTESIAN_POINT ( 'NONE',  ( -32.50000000000000000, -120.0000000000000000, -2.500000000000000000 ) ) ;
#34390=CARTESIAN_POINT ( 'NONE',  ( -70.53423027509626309, -217.0820393249940423, -5.500000000000000000 ) ) ;
#34400=CARTESIAN_POINT ( 'NONE',  ( 0.000000000000000000, 0.000000000000000000, -5.500000000000000000 ) ) ;
#34405=FACE_OUTER_BOUND ( 'NONE', #18805, .T. ) ;
#34418=ORIENTED_EDGE ( 'NONE', *, *, #5988, .F. ) ;
#34422=AXIS2_PLACEMENT_3D ( 'NONE', #26465, #34272, #31359 ) ;
#34426=CARTESIAN_POINT ( 'NONE',  ( 14.59956846177685996, -138.4757300459248484, 5.500000000000000000 ) ) ;
#34458=AXIS2_PLACEMENT_3D ( 'NONE', #33984, #12217, #30558 ) ;
#34462=LINE ( 'NONE', #30336, #36344 ) ;
#34473=FILL_AREA_STYLE_COLOUR ( '', #28825 ) ;
#34479=UNCERTAINTY_MEASURE_WITH_UNIT (LENGTH_MEASURE( 1.000000000000000082E-05 ), #37118, 'distance_accuracy_value', 'NONE');
#34484=PLANE ( 'NONE',  #8860 ) ;
#34508=CARTESIAN_POINT ( 'NONE',  ( 22.08297821871651578, -111.8242998470044540, -2.500000000000000000 ) ) ;
#34517=CARTESIAN_POINT ( 'NONE',  ( 1.029419772574596825, -118.9089936151275140, -2.500000000000000000 ) ) ;
#34518=AXIS2_PLACEMENT_3D ( 'NONE', #9837, #5689, #16944 ) ;
#34522=ADVANCED_FACE ( 'NONE', ( #29369 ), #14687, .F. ) ;
#34523=AXIS2_PLACEMENT_3D ( 'NONE', #23580, #35577, #20156 ) ;
#34525=VECTOR ( 'NONE', #29306, 1000.000000000000000 ) ;
#34545=VERTEX_POINT ( 'NONE', #47956 ) ;
#34548=LINE ( 'NONE', #42398, #42590 ) ;
#34550=VECTOR ( 'NONE', #31973, 1000.000000000000227 ) ;
#34557=EDGE_CURVE ( 'NONE', #9209, #35598, #10770, .T. ) ;
#34566=FACE_OUTER_BOUND ( 'NONE', #23203, .T. ) ;
#34576=EDGE_CURVE ( 'NONE', #37461, #3370, #33747, .T. ) ;
#34591=DIRECTION ( 'NONE',  ( -0.8541291221503261033, 0.5200609990133016058, 0.000000000000000000 ) ) ;
#34603=ORIENTED_EDGE ( 'NONE', *, *, #9300, .F. ) ;
#34621=LINE ( 'NONE', #1105, #6939 ) ;
#34628=DIRECTION ( 'NONE',  ( -0.02332147558787674158, -0.9997280174009349762, 0.000000000000000000 ) ) ;
#34634=LINE ( 'NONE', #38093, #13607 ) ;
#34645=EDGE_LOOP ( 'NONE', ( #39905, #42286, #10872, #47941 ) ) ;
#34652=CARTESIAN_POINT ( 'NONE',  ( 114.1267819554180392, -82.91796067500511924, 5.500000000000000000 ) ) ;
#34680=AXIS2_PLACEMENT_3D ( 'NONE', #20397, #16980, #42199 ) ;
#34692=VECTOR ( 'NONE', #23337, 1000.000000000000000 ) ;
#34710=ORIENTED_EDGE ( 'NONE', *, *, #47124, .T. ) ;
#34714=LINE ( 'NONE', #30826, #11278 ) ;
#34735=VERTEX_POINT ( 'NONE', #4870 ) ;
#34761=DIRECTION ( 'NONE',  ( -0.000000000000000000, 0.000000000000000000, -1.000000000000000000 ) ) ;
#34762=AXIS2_PLACEMENT_3D ( 'NONE', #45256, #37666, #22262 ) ;
#34768=DIRECTION ( 'NONE',  ( 0.3853207896976523772, -0.9227826878668550226, 0.000000000000000000 ) ) ;
#34772=LINE ( 'NONE', #38452, #13633 ) ;
#34803=ORIENTED_EDGE ( 'NONE', *, *, #9174, .F. ) ;
#34813=CARTESIAN_POINT ( 'NONE',  ( 12.50000000000000000, -107.5000000000000000, 2.500000000000000000 ) ) ;
#34816=VECTOR ( 'NONE', #33869, 1000.000000000000000 ) ;
#34828=ORIENTED_EDGE ( 'NONE', *, *, #8602, .F. ) ;
#34834=CARTESIAN_POINT ( 'NONE',  ( -19.90058851926621131, -132.5883508287165853, 5.500000000000000000 ) ) ;
#34844=LINE ( 'NONE', #45146, #34025 ) ;
#34851=ORIENTED_EDGE ( 'NONE', *, *, #20846, .T. ) ;
#34852=ORIENTED_EDGE ( 'NONE', *, *, #34926, .T. ) ;
#34853=CARTESIAN_POINT ( 'NONE',  ( -18.12185313557660038, -104.9634299478706794, -5.500000000000000000 ) ) ;
#34855=CIRCLE ( 'NONE', #47381, 30.50000000000000000 ) ;
#34871=CARTESIAN_POINT ( 'NONE',  ( -30.50000000000000000, -120.0000000000000000, -5.500000000000000000 ) ) ;
#34912=DIRECTION ( 'NONE',  ( -0.2867529058022035837, 0.9580045777625452175, 0.000000000000000000 ) ) ;
#34926=EDGE_CURVE ( 'NONE', #4822, #45107, #10950, .T. ) ;
#34939=FACE_OUTER_BOUND ( 'NONE', #3064, .T. ) ;
#34958=CARTESIAN_POINT ( 'NONE',  ( -12.50000000000000000, -132.5000000000000000, -2.500000000000000000 ) ) ;
#34969=PLANE ( 'NONE',  #10602 ) ;
#34981=ORIENTED_EDGE ( 'NONE', *, *, #18913, .T. ) ;
#35003=ORIENTED_EDGE ( 'NONE', *, *, #35037, .T. ) ;
#35013=CARTESIAN_POINT ( 'NONE',  ( -22.17439115976385366, -112.2188447712574799, -2.500000000000000000 ) ) ;
#35031=EDGE_CURVE ( 'NONE', #41733, #13231, #13903, .T. ) ;
#35037=EDGE_CURVE ( 'NONE', #10301, #41947, #36415, .T. ) ;
#35045=ORIENTED_EDGE ( 'NONE', *, *, #28424, .F. ) ;
#35046=CARTESIAN_POINT ( 'NONE',  ( 13.83832728059186046, -142.6495187161941089, 5.500000000000000000 ) ) ;
#35060=FACE_BOUND ( 'NONE', #35937, .T. ) ;
#35061=CARTESIAN_POINT ( 'NONE',  ( 6.377742925735834234, -145.7647898336708181, 5.500000000000000000 ) ) ;
#35086=EDGE_CURVE ( 'NONE', #2942, #37452, #8247, .T. ) ;
#35088=CARTESIAN_POINT ( 'NONE',  ( 12.13205353604972991, -140.1820037904669789, 5.500000000000000000 ) ) ;
#35089=ADVANCED_FACE ( 'NONE', ( #41305 ), #27101, .F. ) ;
#35093=VERTEX_POINT ( 'NONE', #15111 ) ;
#35102=ORIENTED_EDGE ( 'NONE', *, *, #3299, .T. ) ;
#35113=CARTESIAN_POINT ( 'NONE',  ( 20.85212586905262100, -130.9402397935870965, 5.500000000000000000 ) ) ;
#35130=CARTESIAN_POINT ( 'NONE',  ( -1.474095553543409487, -120.2775649455957989, -2.500000000000000000 ) ) ;
#35139=EDGE_CURVE ( 'NONE', #17971, #25651, #33936, .T. ) ;
#35145=EDGE_LOOP ( 'NONE', ( #14777, #21684, #30217, #16165 ) ) ;
#35147=DIRECTION ( 'NONE',  ( 0.000000000000000000, 0.000000000000000000, 1.000000000000000000 ) ) ;
#35158=ORIENTED_EDGE ( 'NONE', *, *, #27522, .F. ) ;
#35170=ORIENTED_EDGE ( 'NONE', *, *, #17179, .F. ) ;
#35178=DIRECTION ( 'NONE',  ( 0.4279312458753000703, 0.9038112904824842087, 0.000000000000000000 ) ) ;
#35179=LINE ( 'NONE', #38880, #42869 ) ;
#35200=EDGE_LOOP ( 'NONE', ( #6673, #11016 ) ) ;
#35213=( NAMED_UNIT ( * ) SI_UNIT ( $, .STERADIAN. ) SOLID_ANGLE_UNIT ( ) );
#35217=CARTESIAN_POINT ( 'NONE',  ( -25.50183398199384754, -112.6408924756582053, 5.500000000000000000 ) ) ;
#35236=EDGE_LOOP ( 'NONE', ( #33495, #21693, #303, #45783 ) ) ;
#35252=EDGE_CURVE ( 'NONE', #41733, #45238, #28059, .T. ) ;
#35257=VERTEX_POINT ( 'NONE', #2113 ) ;
#35260=CARTESIAN_POINT ( 'NONE',  ( -4.653126046682595884, -146.1313684676804314, 2.500000000000000000 ) ) ;
#35263=AXIS2_PLACEMENT_3D ( 'NONE', #40452, #30, #36752 ) ;
#35266=DIRECTION ( 'NONE',  ( 0.7950889364178796992, -0.6064928550163511956, 0.000000000000000000 ) ) ;
#35274=AXIS2_PLACEMENT_3D ( 'NONE', #25660, #11720, #10756 ) ;
#35289=LINE ( 'NONE', #19623, #38346 ) ;
#35291=CARTESIAN_POINT ( 'NONE',  ( 12.13205353604972991, -140.1820037904669789, 5.500000000000000000 ) ) ;
#35301=EDGE_CURVE ( 'NONE', #28791, #10091, #27570, .T. ) ;
#35313=CARTESIAN_POINT ( 'NONE',  ( 21.07894319797337701, -103.8699611390234878, -2.500000000000000444 ) ) ;
#35317=LINE ( 'NONE', #15755, #34692 ) ;
#35323=CARTESIAN_POINT ( 'NONE',  ( -0.4966694826856976608, -121.4153866697721611, -2.500000000000000000 ) ) ;
#35339=VERTEX_POINT ( 'NONE', #25748 ) ;
#35341=AXIS2_PLACEMENT_3D ( 'NONE', #33727, #18568, #41575 ) ;
#35356=DIRECTION ( 'NONE',  ( -0.000000000000000000, -0.000000000000000000, -1.000000000000000000 ) ) ;
#35358=VERTEX_POINT ( 'NONE', #29670 ) ;
#35360=ORIENTED_EDGE ( 'NONE', *, *, #37768, .F. ) ;
#35368=PLANE ( 'NONE',  #31469 ) ;
#35397=VECTOR ( 'NONE', #35975, 1000.000000000000000 ) ;
#35400=CARTESIAN_POINT ( 'NONE',  ( -26.29030328629083968, -123.6496510949466341, 5.500000000000000000 ) ) ;
#35418=ORIENTED_EDGE ( 'NONE', *, *, #41122, .F. ) ;
#35423=CARTESIAN_POINT ( 'NONE',  ( -1.029419772574582836, -121.0910063848724718, 2.500000000000000000 ) ) ;
#35425=ADVANCED_FACE ( 'NONE', ( #29913 ), #37010, .F. ) ;
#35435=ORIENTED_EDGE ( 'NONE', *, *, #47916, .F. ) ;
#35438=VECTOR ( 'NONE', #11662, 1000.000000000000000 ) ;
#35439=VECTOR ( 'NONE', #25963, 1000.000000000000114 ) ;
#35440=AXIS2_PLACEMENT_3D ( 'NONE', #8597, #37269, #3733 ) ;
#35445=VERTEX_POINT ( 'NONE', #33349 ) ;
#35452=CARTESIAN_POINT ( 'NONE',  ( -8.826826895187510402, -94.96827758698185562, 2.500000000000000000 ) ) ;
#35453=CARTESIAN_POINT ( 'NONE',  ( -35.50000000000000711, -120.0000000000000000, 2.500000000000000000 ) ) ;
#35456=VECTOR ( 'NONE', #1520, 1000.000000000000114 ) ;
#35471=ORIENTED_EDGE ( 'NONE', *, *, #40599, .F. ) ;
#35500=CARTESIAN_POINT ( 'NONE',  ( 89.17737905728634473, -39.70432723693593857, 5.500000000000000000 ) ) ;
#35520=ORIENTED_EDGE ( 'NONE', *, *, #48116, .T. ) ;
#35528=AXIS2_PLACEMENT_3D ( 'NONE', #35217, #5137, #42824 ) ;
#35535=DIRECTION ( 'NONE',  ( 0.000000000000000000, 0.000000000000000000, -1.000000000000000000 ) ) ;
#35538=VERTEX_POINT ( 'NONE', #30643 ) ;
#35539=CARTESIAN_POINT ( 'NONE',  ( -7.670864526094549163, -97.73662565058241114, 5.500000000000000000 ) ) ;
#35545=CARTESIAN_POINT ( 'NONE',  ( -23.97194136764370498, -131.3950000906648938, -2.500000000000000444 ) ) ;
#35561=ORIENTED_EDGE ( 'NONE', *, *, #35778, .T. ) ;
#35568=ORIENTED_EDGE ( 'NONE', *, *, #9884, .F. ) ;
#35569=DIRECTION ( 'NONE',  ( 0.7585478161175723821, 0.6516173805718057377, -0.000000000000000000 ) ) ;
#35577=DIRECTION ( 'NONE',  ( 0.08130631524009970801, -0.9966891607226786576, 0.000000000000000000 ) ) ;
#35585=ORIENTED_EDGE ( 'NONE', *, *, #34252, .F. ) ;
#35598=VERTEX_POINT ( 'NONE', #38231 ) ;
#35614=EDGE_CURVE ( 'NONE', #19505, #19471, #17627, .T. ) ;
#35615=ORIENTED_EDGE ( 'NONE', *, *, #9770, .F. ) ;
#35629=LINE ( 'NONE', #2102, #11093 ) ;
#35635=PLANE ( 'NONE',  #15041 ) ;
#35638=DIRECTION ( 'NONE',  ( 0.000000000000000000, 0.000000000000000000, 1.000000000000000000 ) ) ;
#35646=EDGE_CURVE ( 'NONE', #5501, #31423, #47015, .T. ) ;
#35651=EDGE_CURVE ( 'NONE', #25478, #7237, #31872, .T. ) ;
#35664=EDGE_LOOP ( 'NONE', ( #41950, #32826, #38851, #29136 ) ) ;
#35671=EDGE_CURVE ( 'NONE', #2158, #42271, #24253, .T. ) ;
#35674=VERTEX_POINT ( 'NONE', #13246 ) ;
#35676=EDGE_LOOP ( 'NONE', ( #11110, #47982, #32500, #27355 ) ) ;
#35682=CARTESIAN_POINT ( 'NONE',  ( -18.24502636017238899, -100.7225776329765665, -5.500000000000000000 ) ) ;
#35686=ORIENTED_EDGE ( 'NONE', *, *, #25728, .F. ) ;
#35688=AXIS2_PLACEMENT_3D ( 'NONE', #23766, #6137, #1998 ) ;
#35695=CARTESIAN_POINT ( 'NONE',  ( -18.12185313557660038, -104.9634299478706794, 5.500000000000000000 ) ) ;
#35698=CARTESIAN_POINT ( 'NONE',  ( -16.07206065793331007, -141.0698568150738197, 2.500000000000000000 ) ) ;
#35711=EDGE_CURVE ( 'NONE', #6288, #5501, #27368, .T. ) ;
#35730=CARTESIAN_POINT ( 'NONE',  ( 25.81725066941077529, -113.8380548628854854, -5.500000000000000000 ) ) ;
#35731=EDGE_LOOP ( 'NONE', ( #46322, #2344, #31631, #21789 ) ) ;
#35734=FACE_OUTER_BOUND ( 'NONE', #9730, .T. ) ;
#35738=ORIENTED_EDGE ( 'NONE', *, *, #29606, .F. ) ;
#35739=VERTEX_POINT ( 'NONE', #45732 ) ;
#35753=CARTESIAN_POINT ( 'NONE',  ( 12.69589495141918611, -96.69089767102708777, 5.500000000000000000 ) ) ;
#35760=ORIENTED_EDGE ( 'NONE', *, *, #6812, .T. ) ;
#35778=EDGE_CURVE ( 'NONE', #17554, #15896, #35179, .T. ) ;
#35781=CARTESIAN_POINT ( 'NONE',  ( -25.50183398199384754, -112.6408924756582053, -5.500000000000000000 ) ) ;
#35792=CARTESIAN_POINT ( 'NONE',  ( -7.670864526094549163, -97.73662565058241114, -5.500000000000000000 ) ) ;
#35795=ORIENTED_EDGE ( 'NONE', *, *, #27612, .F. ) ;
#35804=CARTESIAN_POINT ( 'NONE',  ( -0.9774260708577104939, -118.8621782758236378, 2.500000000000000000 ) ) ;
#35812=DIRECTION ( 'NONE',  ( -0.9435911131814395114, 0.3311129884571304971, 0.000000000000000000 ) ) ;
#35816=LINE ( 'NONE', #13796, #43193 ) ;
#35817=CARTESIAN_POINT ( 'NONE',  ( 26.09152095774781799, -124.8716048804687375, 5.500000000000000000 ) ) ;
#35836=CARTESIAN_POINT ( 'NONE',  ( -20.30386590532152979, -102.9045904027214959, 5.500000000000000000 ) ) ;
#35837=CARTESIAN_POINT ( 'NONE',  ( -7.670864526094549163, -97.73662565058241114, 2.500000000000000000 ) ) ;
#35838=ORIENTED_EDGE ( 'NONE', *, *, #14700, .F. ) ;
#35858=DIRECTION ( 'NONE',  ( -0.9227826878668540234, -0.3853207896976546531, 0.000000000000000000 ) ) ;
#35859=LINE ( 'NONE', #36101, #34550 ) ;
#35866=DIRECTION ( 'NONE',  ( 0.000000000000000000, -0.000000000000000000, 1.000000000000000000 ) ) ;
#35867=DIRECTION ( 'NONE',  ( -0.2306669878475648139, -0.9730327541852491491, 0.000000000000000000 ) ) ;
#35875=EDGE_LOOP ( 'NONE', ( #25853, #22231, #35615, #44984 ) ) ;
#35885=ORIENTED_EDGE ( 'NONE', *, *, #17642, .F. ) ;
#35919=CARTESIAN_POINT ( 'NONE',  ( -24.50849501662245800, -109.8101191361138831, 5.500000000000000000 ) ) ;
#35923=DIRECTION ( 'NONE',  ( 0.9227826878668540234, 0.3853207896976547087, 0.000000000000000000 ) ) ;
#35928=LINE ( 'NONE', #35453, #7312 ) ;
#35937=EDGE_LOOP ( 'NONE', ( #31039, #34091, #45016, #41879 ) ) ;
#35957=ORIENTED_EDGE ( 'NONE', *, *, #27421, .T. ) ;
#35975=DIRECTION ( 'NONE',  ( -0.000000000000000000, -0.000000000000000000, -1.000000000000000000 ) ) ;
#35987=CARTESIAN_POINT ( 'NONE',  ( -19.90058851926621131, -132.5883508287165853, -5.500000000000000000 ) ) ;
#36002=FACE_OUTER_BOUND ( 'NONE', #16093, .T. ) ;
#36013=ORIENTED_EDGE ( 'NONE', *, *, #160, .F. ) ;
#36014=ORIENTED_EDGE ( 'NONE', *, *, #30718, .T. ) ;
#36040=VECTOR ( 'NONE', #4395, 1000.000000000000000 ) ;
#36041=DIRECTION ( 'NONE',  ( -0.6064928550163524168, -0.7950889364178789220, 0.000000000000000000 ) ) ;
#36043=EDGE_LOOP ( 'NONE', ( #27722, #14633, #46256, #3269 ) ) ;
#36080=EDGE_CURVE ( 'NONE', #47237, #41733, #5615, .T. ) ;
#36101=CARTESIAN_POINT ( 'NONE',  ( 26.28306158492127764, -123.3838844133976522, -2.500000000000000000 ) ) ;
#36123=FACE_OUTER_BOUND ( 'NONE', #23414, .T. ) ;
#36124=ORIENTED_EDGE ( 'NONE', *, *, #21495, .F. ) ;
#36142=ORIENTED_EDGE ( 'NONE', *, *, #8243, .F. ) ;
#36147=FACE_BOUND ( 'NONE', #27822, .T. ) ;
#36150=LINE ( 'NONE', #21943, #39087 ) ;
#36162=DIRECTION ( 'NONE',  ( -0.7950889364178796992, 0.6064928550163511956, 0.000000000000000000 ) ) ;
#36185=CARTESIAN_POINT ( 'NONE',  ( 19.12409105625795291, -101.5943176906707919, -5.500000000000000000 ) ) ;
#36206=ORIENTED_EDGE ( 'NONE', *, *, #44137, .F. ) ;
#36218=CARTESIAN_POINT ( 'NONE',  ( -6.880223345695647197, -142.5202692415819854, -5.500000000000000000 ) ) ;
#36220=CARTESIAN_POINT ( 'NONE',  ( -23.97194136764370498, -131.3950000906648938, 5.500000000000000000 ) ) ;
#36228=CARTESIAN_POINT ( 'NONE',  ( 30.50000000000000000, -120.0000000000000000, 2.500000000000000000 ) ) ;
#36252=ORIENTED_EDGE ( 'NONE', *, *, #38416, .F. ) ;
#36260=FACE_OUTER_BOUND ( 'NONE', #38794, .T. ) ;
#36266=ADVANCED_FACE ( 'NONE', ( #41085 ), #41317, .T. ) ;
#36276=ORIENTED_EDGE ( 'NONE', *, *, #19375, .T. ) ;
#36286=LINE ( 'NONE', #46833, #45428 ) ;
#36288=ADVANCED_FACE ( 'NONE', ( #41803 ), #18775, .F. ) ;
#36314=EDGE_LOOP ( 'NONE', ( #2739, #4660, #42065, #37910 ) ) ;
#36328=CARTESIAN_POINT ( 'NONE',  ( 1.233757462863572574, -119.1468631277289347, -2.500000000000000000 ) ) ;
#36344=VECTOR ( 'NONE', #48432, 1000.000000000000114 ) ;
#36350=ADVANCED_FACE ( 'NONE', ( #41551 ), #8262, .F. ) ;
#36352=DIRECTION ( 'NONE',  ( 0.6516173805718079581, -0.7585478161175704948, 0.000000000000000000 ) ) ;
#36390=ORIENTED_EDGE ( 'NONE', *, *, #28562, .F. ) ;
#36394=DIRECTION ( 'NONE',  ( -0.9827303690289279636, -0.1850432970638682117, 0.000000000000000000 ) ) ;
#36404=VERTEX_POINT ( 'NONE', #23666 ) ;
#36415=LINE ( 'NONE', #47652, #20114 ) ;
#36420=DIRECTION ( 'NONE',  ( -0.02332147558787823691, -0.9997280174009349762, 0.000000000000000000 ) ) ;
#36423=EDGE_CURVE ( 'NONE', #37836, #47237, #1639, .T. ) ;
#36428=VECTOR ( 'NONE', #7866, 1000.000000000000000 ) ;
#36433=EDGE_CURVE ( 'NONE', #32597, #13263, #27117, .T. ) ;
#36445=DIRECTION ( 'NONE',  ( 1.000000000000000000, 0.000000000000000000, 0.000000000000000000 ) ) ;
#36463=CARTESIAN_POINT ( 'NONE',  ( 23.41451323550360186, -132.5004227906269989, 5.500000000000000000 ) ) ;
#36474=CARTESIAN_POINT ( 'NONE',  ( -16.06301359042743115, -102.7814171781257357, 5.500000000000000000 ) ) ;
#36477=EDGE_CURVE ( 'NONE', #9793, #29613, #4827, .T. ) ;
#36491=DIRECTION ( 'NONE',  ( 0.2867529058022035837, -0.9580045777625452175, 0.000000000000000000 ) ) ;
#36496=CARTESIAN_POINT ( 'NONE',  ( 35.50000000000000711, -120.0000000000000000, -5.500000000000000000 ) ) ;
#36555=DIRECTION ( 'NONE',  ( -0.9827303690289279636, -0.1850432970638682117, 0.000000000000000000 ) ) ;
#36556=DIRECTION ( 'NONE',  ( -0.3853207896976523772, 0.9227826878668550226, 0.000000000000000000 ) ) ;
#36560=ORIENTED_EDGE ( 'NONE', *, *, #23426, .T. ) ;
#36565=ORIENTED_EDGE ( 'NONE', *, *, #7779, .T. ) ;
#36577=PLANE ( 'NONE',  #40936 ) ;
#36582=LINE ( 'NONE', #37313, #17333 ) ;
#36595=VECTOR ( 'NONE', #43584, 1000.000000000000000 ) ;
#36604=ORIENTED_EDGE ( 'NONE', *, *, #25728, .T. ) ;
#36626=CARTESIAN_POINT ( 'NONE',  ( -18.24502636017238899, -100.7225776329765665, 5.500000000000000000 ) ) ;
#36627=FACE_BOUND ( 'NONE', #24602, .T. ) ;
#36634=DIRECTION ( 'NONE',  ( -0.000000000000000000, -0.000000000000000000, 1.000000000000000000 ) ) ;
#36635=ADVANCED_FACE ( 'NONE', ( #36123 ), #24870, .F. ) ;
#36637=ORIENTED_EDGE ( 'NONE', *, *, #187, .T. ) ;
#36638=CARTESIAN_POINT ( 'NONE',  ( 1.384174031800307736, -119.4220188154534981, -2.500000000000000000 ) ) ;
#36650=PLANE ( 'NONE',  #30794 ) ;
#36656=VECTOR ( 'NONE', #20468, 1000.000000000000114 ) ;
#36657=AXIS2_PLACEMENT_3D ( 'NONE', #23399, #37853, #11913 ) ;
#36683=CARTESIAN_POINT ( 'NONE',  ( 23.11608002360578240, -124.4885236261218182, 5.500000000000000000 ) ) ;
#36687=CARTESIAN_POINT ( 'NONE',  ( 12.69589495141918611, -96.69089767102708777, 5.500000000000000000 ) ) ;
#36710=VERTEX_POINT ( 'NONE', #370 ) ;
#36713=VECTOR ( 'NONE', #40311, 1000.000000000000114 ) ;
#36716=DIRECTION ( 'NONE',  ( -0.000000000000000000, -0.000000000000000000, -1.000000000000000000 ) ) ;
#36723=PLANE ( 'NONE',  #2349 ) ;
#36729=DIRECTION ( 'NONE',  ( -0.000000000000000000, -0.000000000000000000, -1.000000000000000000 ) ) ;
#36733=VERTEX_POINT ( 'NONE', #8201 ) ;
#36744=PLANE ( 'NONE',  #39277 ) ;
#36749=PLANE ( 'NONE',  #33648 ) ;
#36752=DIRECTION ( 'NONE',  ( -0.7585478161175716050, -0.6516173805718067369, 0.000000000000000000 ) ) ;
#36767=LINE ( 'NONE', #22575, #47548 ) ;
#36776=LINE ( 'NONE', #14275, #12020 ) ;
#36783=VECTOR ( 'NONE', #44651, 1000.000000000000000 ) ;
#36794=AXIS2_PLACEMENT_3D ( 'NONE', #29646, #26227, #41169 ) ;
#36801=ORIENTED_EDGE ( 'NONE', *, *, #35614, .T. ) ;
#36814=CARTESIAN_POINT ( 'NONE',  ( -23.97194136764370498, -131.3950000906648938, -5.500000000000000000 ) ) ;
#36815=LINE ( 'NONE', #40738, #1738 ) ;
#36820=DIRECTION ( 'NONE',  ( -0.6862798483830533369, -0.7273375899149812085, 0.000000000000000000 ) ) ;
#36822=LINE ( 'NONE', #3288, #1232 ) ;
#36828=ORIENTED_EDGE ( 'NONE', *, *, #8243, .T. ) ;
#36829=CARTESIAN_POINT ( 'NONE',  ( 0.000000000000000000, -120.0000000000000000, 2.500000000000000000 ) ) ;
#36835=VECTOR ( 'NONE', #15411, 1000.000000000000114 ) ;
#36844=EDGE_CURVE ( 'NONE', #14848, #36901, #38281, .T. ) ;
#36851=EDGE_LOOP ( 'NONE', ( #32498, #29879, #12263, #5890 ) ) ;
#36856=FACE_BOUND ( 'NONE', #2962, .T. ) ;
#36858=VERTEX_POINT ( 'NONE', #10064 ) ;
#36881=DIRECTION ( 'NONE',  ( -0.3311129884571281101, -0.9435911131814402886, 0.000000000000000000 ) ) ;
#36897=ORIENTED_EDGE ( 'NONE', *, *, #47320, .T. ) ;
#36898=ADVANCED_FACE ( 'NONE', ( #36002 ), #28675, .F. ) ;
#36901=VERTEX_POINT ( 'NONE', #34365 ) ;
#36930=CIRCLE ( 'NONE', #33023, 30.50000000000000000 ) ;
#36943=ORIENTED_EDGE ( 'NONE', *, *, #18464, .T. ) ;
#36944=UNCERTAINTY_MEASURE_WITH_UNIT (LENGTH_MEASURE( 1.000000000000000082E-05 ), #46490, 'distance_accuracy_value', 'NONE');
#36951=EDGE_CURVE ( 'NONE', #42762, #28234, #6639, .T. ) ;
#36963=EDGE_LOOP ( 'NONE', ( #29760, #6893, #6889, #4673 ) ) ;
#36966=PRODUCT_DEFINITION ( 'UNKNOWN', '', #13934, #44784 ) ;
#36979=DIRECTION ( 'NONE',  ( 0.6516173805718078471, -0.7585478161175706058, 0.000000000000000000 ) ) ;
#36984=EDGE_LOOP ( 'NONE', ( #14270, #25469, #44682, #6430 ) ) ;
#36994=AXIS2_PLACEMENT_3D ( 'NONE', #48220, #11267, #7593 ) ;
#37010=PLANE ( 'NONE',  #31912 ) ;
#37013=AXIS2_PLACEMENT_3D ( 'NONE', #28056, #9432, #35867 ) ;
#37021=AXIS2_PLACEMENT_3D ( 'NONE', #46741, #9044, #16875 ) ;
#37025=AXIS2_PLACEMENT_3D ( 'NONE', #2780, #18437, #21377 ) ;
#37036=CARTESIAN_POINT ( 'NONE',  ( -12.50000000000000000, -132.5000000000000000, 2.500000000000000000 ) ) ;
#37039=LINE ( 'NONE', #44626, #16030 ) ;
#37044=LINE ( 'NONE', #3514, #46461 ) ;
#37064=DIRECTION ( 'NONE',  ( -0.000000000000000000, -0.000000000000000000, -1.000000000000000000 ) ) ;
#37065=FACE_OUTER_BOUND ( 'NONE', #30419, .T. ) ;
#37073=DIRECTION ( 'NONE',  ( 0.9997280174009348652, -0.02332147558787931590, 0.000000000000000000 ) ) ;
#37076=LINE ( 'NONE', #6744, #10487 ) ;
#37078=CARTESIAN_POINT ( 'NONE',  ( 16.84844760790522855, -103.5491698323862124, 5.500000000000000000 ) ) ;
#37101=ORIENTED_EDGE ( 'NONE', *, *, #45302, .T. ) ;
#37102=EDGE_LOOP ( 'NONE', ( #23943, #4652, #40535, #13175 ) ) ;
#37118=( LENGTH_UNIT ( ) NAMED_UNIT ( * ) SI_UNIT ( .MILLI., .METRE. ) );
#37123=VECTOR ( 'NONE', #17981, 1000.000000000000000 ) ;
#37135=CIRCLE ( 'NONE', #48065, 35.50000000000000711 ) ;
#37151=ORIENTED_EDGE ( 'NONE', *, *, #1456, .T. ) ;
#37155=EDGE_LOOP ( 'NONE', ( #10611, #48281, #38789, #46991 ) ) ;
#37179=ORIENTED_EDGE ( 'NONE', *, *, #10469, .T. ) ;
#37187=LINE ( 'NONE', #26176, #36835 ) ;
#37196=AXIS2_PLACEMENT_3D ( 'NONE', #47539, #43636, #42923 ) ;
#37206=VECTOR ( 'NONE', #37557, 1000.000000000000114 ) ;
#37232=CARTESIAN_POINT ( 'NONE',  ( -21.67772167707813935, -110.8034581014852762, 5.500000000000000000 ) ) ;
#37242=DIRECTION ( 'NONE',  ( 0.6064928550163511956, 0.7950889364178798102, -0.000000000000000000 ) ) ;
#37245=DIRECTION ( 'NONE',  ( -0.8541291221503266584, 0.5200609990133008287, 0.000000000000000000 ) ) ;
#37259=ADVANCED_FACE ( 'NONE', ( #13203 ), #28128, .F. ) ;
#37269=DIRECTION ( 'NONE',  ( -0.2306669878475622604, -0.9730327541852497042, 0.000000000000000000 ) ) ;
#37284=CARTESIAN_POINT ( 'NONE',  ( 22.94323693612312809, -114.6983135802921083, 5.500000000000000000 ) ) ;
#37289=DIRECTION ( 'NONE',  ( -0.08130631524010122069, 0.9966891607226784355, 0.000000000000000000 ) ) ;
#37295=DIRECTION ( 'NONE',  ( 0.9227826878668540234, 0.3853207896976547087, 0.000000000000000000 ) ) ;
#37298=VERTEX_POINT ( 'NONE', #27914 ) ;
#37304=LINE ( 'NONE', #33618, #8987 ) ;
#37313=CARTESIAN_POINT ( 'NONE',  ( 21.85433023846371370, -135.0628101570779620, 5.500000000000000000 ) ) ;
#37332=VECTOR ( 'NONE', #7624, 1000.000000000000000 ) ;
#37339=CARTESIAN_POINT ( 'NONE',  ( -25.00516449930816876, -111.2255058058861010, -2.500000000000000000 ) ) ;
#37345=EDGE_LOOP ( 'NONE', ( #20966, #35471, #32757, #4427 ) ) ;
#37351=FACE_BOUND ( 'NONE', #48257, .T. ) ;
#37360=CARTESIAN_POINT ( 'NONE',  ( -6.880223345695647197, -142.5202692415819854, 5.500000000000000000 ) ) ;
#37370=ORIENTED_EDGE ( 'NONE', *, *, #25689, .F. ) ;
#37385=CARTESIAN_POINT ( 'NONE',  ( -18.12185313557660038, -104.9634299478706794, 5.500000000000000000 ) ) ;
#37392=ORIENTED_EDGE ( 'NONE', *, *, #3796, .T. ) ;
#37394=CARTESIAN_POINT ( 'NONE',  ( 1.355716935723751293, -120.6418968688129496, 2.500000000000000000 ) ) ;
#37397=ADVANCED_FACE ( 'NONE', ( #32993 ), #47917, .F. ) ;
#37405=ADVANCED_FACE ( 'NONE', ( #29571 ), #18056, .F. ) ;
#37406=DIRECTION ( 'NONE',  ( 0.8541291221503261033, -0.5200609990133016058, 0.000000000000000000 ) ) ;
#37421=FACE_OUTER_BOUND ( 'NONE', #18257, .T. ) ;
#37446=EDGE_CURVE ( 'NONE', #19570, #2942, #13688, .T. ) ;
#37452=VERTEX_POINT ( 'NONE', #36185 ) ;
#37461=VERTEX_POINT ( 'NONE', #24934 ) ;
#37487=DIRECTION ( 'NONE',  ( 0.9730327541852493711, -0.2306669878475637314, 0.000000000000000000 ) ) ;
#37488=DIRECTION ( 'NONE',  ( 0.9827303690289282967, 0.1850432970638667407, -0.000000000000000000 ) ) ;
#37535=VERTEX_POINT ( 'NONE', #30311 ) ;
#37547=LINE ( 'NONE', #21886, #36783 ) ;
#37549=DIRECTION ( 'NONE',  ( -0.1850432970638682395, 0.9827303690289280746, 0.000000000000000000 ) ) ;
#37557=DIRECTION ( 'NONE',  ( -0.9827303690289279636, -0.1850432970638682117, 0.000000000000000000 ) ) ;
#37562=DIRECTION ( 'NONE',  ( -0.000000000000000000, -0.000000000000000000, -1.000000000000000000 ) ) ;
#37579=VECTOR ( 'NONE', #6904, 1000.000000000000000 ) ;
#37603=CARTESIAN_POINT ( 'NONE',  ( 0.000000000000000000, -120.0000000000000000, 2.500000000000000000 ) ) ;
#37610=EDGE_LOOP ( 'NONE', ( #12859, #25002, #37828, #38598 ) ) ;
#37616=DIRECTION ( 'NONE',  ( -0.9997280174009349762, 0.02332147558787671729, 0.000000000000000000 ) ) ;
#37627=LINE ( 'NONE', #46614, #8912 ) ;
#37648=CARTESIAN_POINT ( 'NONE',  ( 23.41451323550360186, -132.5004227906269989, 5.500000000000000000 ) ) ;
#37666=DIRECTION ( 'NONE',  ( 0.9966891607226785466, 0.08130631524010119293, -0.000000000000000000 ) ) ;
#37673=AXIS2_PLACEMENT_3D ( 'NONE', #6975, #21665, #36820 ) ;
#37681=CARTESIAN_POINT ( 'NONE',  ( -25.50183398199384044, -112.6408924756582053, -2.500000000000000000 ) ) ;
#37703=ORIENTED_EDGE ( 'NONE', *, *, #20210, .F. ) ;
#37711=VERTEX_POINT ( 'NONE', #45959 ) ;
#37717=EDGE_LOOP ( 'NONE', ( #28101, #20837, #23142, #4772 ) ) ;
#37721=ORIENTED_EDGE ( 'NONE', *, *, #41303, .F. ) ;
#37730=CARTESIAN_POINT ( 'NONE',  ( -8.826826895187510402, -94.96827758698185562, 5.500000000000000000 ) ) ;
#37746=ORIENTED_EDGE ( 'NONE', *, *, #44001, .F. ) ;
#37758=VECTOR ( 'NONE', #13553, 1000.000000000000000 ) ;
#37759=LINE ( 'NONE', #15259, #28505 ) ;
#37768=EDGE_CURVE ( 'NONE', #28440, #43899, #1642, .T. ) ;
#37779=LINE ( 'NONE', #4267, #14536 ) ;
#37787=VECTOR ( 'NONE', #42026, 1000.000000000000000 ) ;
#37789=CARTESIAN_POINT ( 'NONE',  ( 25.38712131070745315, -112.4010479962415872, 2.500000000000000000 ) ) ;
#37790=FACE_OUTER_BOUND ( 'NONE', #12552, .T. ) ;
#37792=AXIS2_PLACEMENT_3D ( 'NONE', #19385, #19863, #15974 ) ;
#37800=CARTESIAN_POINT ( 'NONE',  ( 23.41451323550360186, -132.5004227906269989, 5.500000000000000000 ) ) ;
#37811=ORIENTED_EDGE ( 'NONE', *, *, #14208, .F. ) ;
#37815=VECTOR ( 'NONE', #10204, 1000.000000000000114 ) ;
#37822=LINE ( 'NONE', #23136, #18723 ) ;
#37828=ORIENTED_EDGE ( 'NONE', *, *, #35086, .T. ) ;
#37836=VERTEX_POINT ( 'NONE', #29277 ) ;
#37847=( NAMED_UNIT ( * ) SI_UNIT ( $, .STERADIAN. ) SOLID_ANGLE_UNIT ( ) );
#37853=DIRECTION ( 'NONE',  ( -0.2306669878475622604, -0.9730327541852497042, 0.000000000000000000 ) ) ;
#37891=FACE_OUTER_BOUND ( 'NONE', #3504, .T. ) ;
#37910=ORIENTED_EDGE ( 'NONE', *, *, #21260, .T. ) ;
#37921=LINE ( 'NONE', #19306, #38301 ) ;
#37931=DIRECTION ( 'NONE',  ( -0.000000000000000000, -0.000000000000000000, -1.000000000000000000 ) ) ;
#37943=AXIS2_PLACEMENT_3D ( 'NONE', #23268, #42111, #26951 ) ;
#37948=VECTOR ( 'NONE', #38665, 1000.000000000000114 ) ;
#37957=EDGE_CURVE ( 'NONE', #25651, #45129, #37822, .T. ) ;
#37963=EDGE_LOOP ( 'NONE', ( #4675, #38625, #25431, #20351 ) ) ;
#37985=CARTESIAN_POINT ( 'NONE',  ( -4.653126046682595884, -146.1313684676804314, 5.500000000000000000 ) ) ;
#37996=EDGE_LOOP ( 'NONE', ( #5010, #9982, #8447, #38507 ) ) ;
#38006=ORIENTED_EDGE ( 'NONE', *, *, #22021, .F. ) ;
#38036=PLANE ( 'NONE',  #18771 ) ;
#38054=DIRECTION ( 'NONE',  ( 0.3311129884571304971, 0.9435911131814395114, -0.000000000000000000 ) ) ;
#38056=VECTOR ( 'NONE', #46722, 1000.000000000000000 ) ;
#38062=VECTOR ( 'NONE', #34912, 1000.000000000000000 ) ;
#38077=ORIENTED_EDGE ( 'NONE', *, *, #29393, .T. ) ;
#38089=ADVANCED_FACE ( 'NONE', ( #42460 ), #16041, .F. ) ;
#38091=CARTESIAN_POINT ( 'NONE',  ( -7.670864526094549163, -97.73662565058241114, 5.500000000000000000 ) ) ;
#38093=CARTESIAN_POINT ( 'NONE',  ( -3.961125083139900749, -143.2122702051246677, 5.500000000000000000 ) ) ;
#38097=CARTESIAN_POINT ( 'NONE',  ( -26.53422223201112828, -120.6595836127786043, -5.500000000000000000 ) ) ;
#38100=VECTOR ( 'NONE', #47602, 1000.000000000000000 ) ;
#38106=LINE ( 'NONE', #23400, #20711 ) ;
#38108=PLANE ( 'NONE',  #44802 ) ;
#38110=DIRECTION ( 'NONE',  ( -0.000000000000000000, -0.000000000000000000, -1.000000000000000000 ) ) ;
#38121=ORIENTED_EDGE ( 'NONE', *, *, #30718, .F. ) ;
#38125=VECTOR ( 'NONE', #14451, 1000.000000000000000 ) ;
#38140=EDGE_CURVE ( 'NONE', #7713, #30905, #5497, .T. ) ;
#38143=ORIENTED_EDGE ( 'NONE', *, *, #3297, .F. ) ;
#38147=DIRECTION ( 'NONE',  ( 0.9038112904824853189, -0.4279312458752977388, 0.000000000000000000 ) ) ;
#38166=VERTEX_POINT ( 'NONE', #34871 ) ;
#38167=CARTESIAN_POINT ( 'NONE',  ( -1.029419772574582836, -121.0910063848724718, -2.500000000000000000 ) ) ;
#38170=LINE ( 'NONE', #222, #20965 ) ;
#38172=EDGE_LOOP ( 'NONE', ( #11827, #44852, #25365, #8937 ) ) ;
#38176=EDGE_LOOP ( 'NONE', ( #42203, #7228, #34033, #8481 ) ) ;
#38186=ORIENTED_EDGE ( 'NONE', *, *, #43357, .T. ) ;
#38205=DIRECTION ( 'NONE',  ( -0.000000000000000000, -0.000000000000000000, -1.000000000000000000 ) ) ;
#38209=DIRECTION ( 'NONE',  ( -0.9997280174009349762, 0.02332147558787674504, 0.000000000000000000 ) ) ;
#38212=CARTESIAN_POINT ( 'NONE',  ( -35.50000000000000711, -120.0000000000000000, -5.500000000000000000 ) ) ;
#38222=CARTESIAN_POINT ( 'NONE',  ( -26.29030328629083968, -123.6496510949466341, 5.500000000000000000 ) ) ;
#38224=DIRECTION ( 'NONE',  ( -1.000000000000000000, 0.000000000000000000, 0.000000000000000000 ) ) ;
#38227=VERTEX_POINT ( 'NONE', #6001 ) ;
#38231=CARTESIAN_POINT ( 'NONE',  ( 12.50000000000000000, -132.5000000000000000, 2.500000000000000000 ) ) ;
#38239=EDGE_CURVE ( 'NONE', #16956, #24649, #24824, .T. ) ;
#38252=CARTESIAN_POINT ( 'NONE',  ( 2.047646702416564768, -96.54137380445985173, 5.500000000000000000 ) ) ;
#38253=DIRECTION ( 'NONE',  ( -0.9966891607226786576, -0.08130631524009861166, 0.000000000000000000 ) ) ;
#38271=DIRECTION ( 'NONE',  ( 0.9918136447140101231, -0.1276937514489694114, 0.000000000000000000 ) ) ;
#38281=CIRCLE ( 'NONE', #6245, 32.50000000000000000 ) ;
#38301=VECTOR ( 'NONE', #30570, 1000.000000000000000 ) ;
#38316=ADVANCED_FACE ( 'NONE', ( #21858 ), #40001, .F. ) ;
#38328=CARTESIAN_POINT ( 'NONE',  ( -24.50849501662245800, -109.8101191361138831, -5.500000000000000000 ) ) ;
#38335=ORIENTED_EDGE ( 'NONE', *, *, #20683, .F. ) ;
#38346=VECTOR ( 'NONE', #15731, 1000.000000000000000 ) ;
#38348=ADVANCED_FACE ( 'NONE', ( #18439 ), #33372, .T. ) ;
#38360=ADVANCED_FACE ( 'NONE', ( #22361 ), #7664, .F. ) ;
#38363=ORIENTED_EDGE ( 'NONE', *, *, #19320, .F. ) ;
#38374=CARTESIAN_POINT ( 'NONE',  ( -16.06301359042743115, -102.7814171781257357, 2.500000000000000000 ) ) ;
#38389=ORIENTED_EDGE ( 'NONE', *, *, #41011, .T. ) ;
#38399=LINE ( 'NONE', #8766, #47978 ) ;
#38403=DIRECTION ( 'NONE',  ( -0.9730327541852491491, 0.2306669878475648139, 0.000000000000000000 ) ) ;
#38406=LINE ( 'NONE', #38167, #4964 ) ;
#38416=EDGE_CURVE ( 'NONE', #45508, #34545, #3507, .T. ) ;
#38429=ORIENTED_EDGE ( 'NONE', *, *, #19177, .T. ) ;
#38452=CARTESIAN_POINT ( 'NONE',  ( -16.06301359042743115, -102.7814171781257357, -5.500000000000000000 ) ) ;
#38457=LINE ( 'NONE', #15945, #39042 ) ;
#38459=CARTESIAN_POINT ( 'NONE',  ( 12.13205353604972814, -140.1820037904669789, -2.500000000000000000 ) ) ;
#38462=LINE ( 'NONE', #16669, #42037 ) ;
#38464=CIRCLE ( 'NONE', #32967, 30.50000000000000000 ) ;
#38483=PLANE ( 'NONE',  #37792 ) ;
#38495=ORIENTED_EDGE ( 'NONE', *, *, #23331, .T. ) ;
#38496=DIRECTION ( 'NONE',  ( -0.000000000000000000, -0.000000000000000000, -1.000000000000000000 ) ) ;
#38501=EDGE_CURVE ( 'NONE', #33738, #18614, #35289, .T. ) ;
#38503=DIRECTION ( 'NONE',  ( 0.6516173805718078471, -0.7585478161175706058, 0.000000000000000000 ) ) ;
#38506=CARTESIAN_POINT ( 'NONE',  ( -26.29030328629083968, -123.6496510949466341, 5.500000000000000000 ) ) ;
#38507=ORIENTED_EDGE ( 'NONE', *, *, #8404, .T. ) ;
#38514=CARTESIAN_POINT ( 'NONE',  ( -48.80839716909612491, -10.37454508288793065, 5.500000000000000000 ) ) ;
#38515=AXIS2_PLACEMENT_3D ( 'NONE', #3358, #7762, #36420 ) ;
#38520=CARTESIAN_POINT ( 'NONE',  ( 3.429551818649054340, -146.3199197248623875, 5.500000000000000000 ) ) ;
#38536=VECTOR ( 'NONE', #24127, 1000.000000000000000 ) ;
#38541=CARTESIAN_POINT ( 'NONE',  ( -18.24502636017238899, -100.7225776329765665, -2.500000000000000444 ) ) ;
#38543=EDGE_CURVE ( 'NONE', #6370, #43886, #46570, .T. ) ;
#38550=DIRECTION ( 'NONE',  ( 0.9227826878668540234, 0.3853207896976547087, 0.000000000000000000 ) ) ;
#38561=DIRECTION ( 'NONE',  ( 0.9730327541852497042, -0.2306669878475623159, 0.000000000000000000 ) ) ;
#38568=ORIENTED_EDGE ( 'NONE', *, *, #26185, .T. ) ;
#38581=DIRECTION ( 'NONE',  ( -0.000000000000000000, -0.000000000000000000, -1.000000000000000000 ) ) ;
#38598=ORIENTED_EDGE ( 'NONE', *, *, #3804, .T. ) ;
#38624=LINE ( 'NONE', #42533, #30541 ) ;
#38625=ORIENTED_EDGE ( 'NONE', *, *, #13677, .F. ) ;
#38638=EDGE_LOOP ( 'NONE', ( #4604, #21266, #48310, #1210 ) ) ;
#38642=LINE ( 'NONE', #5105, #47858 ) ;
#38645=EDGE_CURVE ( 'NONE', #34363, #35739, #6170, .T. ) ;
#38648=CARTESIAN_POINT ( 'NONE',  ( 23.49916127795269460, -121.5130826919798039, 5.500000000000000000 ) ) ;
#38651=ORIENTED_EDGE ( 'NONE', *, *, #30304, .F. ) ;
#38652=ADVANCED_FACE ( 'NONE', ( #40185 ), #2478, .F. ) ;
#38665=DIRECTION ( 'NONE',  ( 0.5687579148473743684, -0.8225049752423791993, 0.000000000000000000 ) ) ;
#38670=EDGE_CURVE ( 'NONE', #551, #43487, #14223, .T. ) ;
#38687=VECTOR ( 'NONE', #15690, 1000.000000000000000 ) ;
#38695=EDGE_CURVE ( 'NONE', #14593, #30621, #13757, .T. ) ;
#38703=CARTESIAN_POINT ( 'NONE',  ( 0.000000000000000000, -120.0000000000000000, 2.500000000000000000 ) ) ;
#38717=FACE_OUTER_BOUND ( 'NONE', #27744, .T. ) ;
#38724=DIRECTION ( 'NONE',  ( 0.000000000000000000, 0.000000000000000000, 1.000000000000000000 ) ) ;
#38735=VERTEX_POINT ( 'NONE', #35545 ) ;
#38750=CARTESIAN_POINT ( 'NONE',  ( 24.95699195200416654, -110.9640411295978595, 5.500000000000000000 ) ) ;
#38758=DIRECTION ( 'NONE',  ( -0.1276937514489679404, -0.9918136447140103451, 0.000000000000000000 ) ) ;
#38759=DIRECTION ( 'NONE',  ( -0.1276937514489679404, -0.9918136447140103451, 0.000000000000000000 ) ) ;
#38772=DIRECTION ( 'NONE',  ( 1.000000000000000000, 0.000000000000000000, 0.000000000000000000 ) ) ;
#38779=AXIS2_PLACEMENT_3D ( 'NONE', #7638, #22568, #33808 ) ;
#38789=ORIENTED_EDGE ( 'NONE', *, *, #20173, .T. ) ;
#38794=EDGE_LOOP ( 'NONE', ( #14453, #2525, #27539, #9698 ) ) ;
#38799=ORIENTED_EDGE ( 'NONE', *, *, #11007, .T. ) ;
#38806=CARTESIAN_POINT ( 'NONE',  ( -26.53422223201112828, -120.6595836127786043, -5.500000000000000000 ) ) ;
#38836=DIRECTION ( 'NONE',  ( -0.8774505977381971134, -0.4796670183876317051, 0.000000000000000000 ) ) ;
#38851=ORIENTED_EDGE ( 'NONE', *, *, #35031, .T. ) ;
#38869=DIRECTION ( 'NONE',  ( -0.9966891607226785466, -0.08130631524009969413, 0.000000000000000000 ) ) ;
#38880=CARTESIAN_POINT ( 'NONE',  ( -7.572224309238338336, -145.4393675041377492, 5.500000000000000000 ) ) ;
#38899=LINE ( 'NONE', #27630, #25981 ) ;
#38904=VERTEX_POINT ( 'NONE', #30068 ) ;
#38907=ORIENTED_EDGE ( 'NONE', *, *, #33977, .F. ) ;
#38911=EDGE_CURVE ( 'NONE', #29613, #46719, #8017, .T. ) ;
#38925=EDGE_CURVE ( 'NONE', #41627, #40068, #38624, .T. ) ;
#38929=LINE ( 'NONE', #733, #23920 ) ;
#38931=ORIENTED_EDGE ( 'NONE', *, *, #12554, .F. ) ;
#38939=VECTOR ( 'NONE', #37931, 1000.000000000000000 ) ;
#38957=DIRECTION ( 'NONE',  ( -0.000000000000000000, -0.000000000000000000, -1.000000000000000000 ) ) ;
#38974=EDGE_CURVE ( 'NONE', #37711, #16641, #5817, .T. ) ;
#38977=CARTESIAN_POINT ( 'NONE',  ( 0.000000000000000000, -120.0000000000000000, -2.500000000000000000 ) ) ;
#38978=CARTESIAN_POINT ( 'NONE',  ( 26.09152095774781799, -124.8716048804687375, -5.500000000000000000 ) ) ;
#38980=LINE ( 'NONE', #17649, #46914 ) ;
#38981=LINE ( 'NONE', #17163, #1072 ) ;
#39000=DIRECTION ( 'NONE',  ( -0.8774505977381971134, -0.4796670183876317051, 0.000000000000000000 ) ) ;
#39015=DIRECTION ( 'NONE',  ( -0.000000000000000000, -0.000000000000000000, -1.000000000000000000 ) ) ;
#39034=EDGE_CURVE ( 'NONE', #45238, #7713, #16341, .T. ) ;
#39036=CARTESIAN_POINT ( 'NONE',  ( -6.880223345695647197, -142.5202692415819854, 5.500000000000000000 ) ) ;
#39040=LINE ( 'NONE', #2086, #11408 ) ;
#39042=VECTOR ( 'NONE', #39680, 1000.000000000000000 ) ;
#39045=VECTOR ( 'NONE', #27352, 1000.000000000000227 ) ;
#39058=PLANE ( 'NONE',  #14424 ) ;
#39069=PLANE ( 'NONE',  #41209 ) ;
#39071=CARTESIAN_POINT ( 'NONE',  ( 25.81725066941077529, -113.8380548628854854, -5.500000000000000000 ) ) ;
#39074=CARTESIAN_POINT ( 'NONE',  ( -16.06301359042743115, -102.7814171781257357, 5.500000000000000000 ) ) ;
#39079=EDGE_CURVE ( 'NONE', #7679, #38227, #6530, .T. ) ;
#39081=VECTOR ( 'NONE', #33510, 1000.000000000000227 ) ;
#39087=VECTOR ( 'NONE', #7016, 1000.000000000000114 ) ;
#39111=ORIENTED_EDGE ( 'NONE', *, *, #11412, .F. ) ;
#39124=CARTESIAN_POINT ( 'NONE',  ( 16.30584220631899228, -140.9432449716519784, -5.500000000000000000 ) ) ;
#39125=CARTESIAN_POINT ( 'NONE',  ( 24.95699195200416654, -110.9640411295978595, 2.500000000000000000 ) ) ;
#39143=PLANE ( 'NONE',  #37021 ) ;
#39154=ORIENTED_EDGE ( 'NONE', *, *, #3255, .F. ) ;
#39156=ORIENTED_EDGE ( 'NONE', *, *, #26011, .T. ) ;
#39170=ORIENTED_EDGE ( 'NONE', *, *, #47668, .F. ) ;
#39184=VECTOR ( 'NONE', #35356, 1000.000000000000000 ) ;
#39200=ORIENTED_EDGE ( 'NONE', *, *, #46361, .T. ) ;
#39207=ORIENTED_EDGE ( 'NONE', *, *, #35646, .F. ) ;
#39249=LINE ( 'NONE', #35817, #25299 ) ;
#39251=AXIS2_PLACEMENT_3D ( 'NONE', #25319, #6739, #18218 ) ;
#39274=DIRECTION ( 'NONE',  ( 0.4279312458753000703, 0.9038112904824842087, -0.000000000000000000 ) ) ;
#39277=AXIS2_PLACEMENT_3D ( 'NONE', #18863, #10320, #47754 ) ;
#39315=EDGE_LOOP ( 'NONE', ( #12588, #7358, #46080, #6781 ) ) ;
#39318=VERTEX_POINT ( 'NONE', #19688 ) ;
#39319=VECTOR ( 'NONE', #30623, 1000.000000000000000 ) ;
#39343=CARTESIAN_POINT ( 'NONE',  ( -23.30023580412278505, -123.4057321492263384, 5.500000000000000000 ) ) ;
#39352=EDGE_CURVE ( 'NONE', #23846, #40712, #24114, .T. ) ;
#39366=DIRECTION ( 'NONE',  ( 0.3311129884571281101, 0.9435911131814402886, 0.000000000000000000 ) ) ;
#39379=AXIS2_PLACEMENT_3D ( 'NONE', #36220, #21281, #43576 ) ;
#39385=ORIENTED_EDGE ( 'NONE', *, *, #27575, .F. ) ;
#39394=FACE_OUTER_BOUND ( 'NONE', #3720, .T. ) ;
#39402=EDGE_LOOP ( 'NONE', ( #3314, #27462, #39156, #48087 ) ) ;
#39408=DIRECTION ( 'NONE',  ( 0.7273375899149812085, -0.6862798483830533369, 0.000000000000000000 ) ) ;
#39420=LINE ( 'NONE', #46996, #25864 ) ;
#39444=EDGE_LOOP ( 'NONE', ( #744, #14492, #1892, #29443 ) ) ;
#39464=AXIS2_PLACEMENT_3D ( 'NONE', #7322, #41354, #3655 ) ;
#39491=ORIENTED_EDGE ( 'NONE', *, *, #5988, .T. ) ;
#39498=CARTESIAN_POINT ( 'NONE',  ( 2.047646702416564768, -96.54137380445985173, 5.500000000000000000 ) ) ;
#39502=DIRECTION ( 'NONE',  ( -0.3853207896976533764, 0.9227826878668546895, 0.000000000000000000 ) ) ;
#39509=VECTOR ( 'NONE', #35812, 1000.000000000000000 ) ;
#39514=CARTESIAN_POINT ( 'NONE',  ( -21.67772167707813935, -110.8034581014852762, 5.500000000000000000 ) ) ;
#39538=ORIENTED_EDGE ( 'NONE', *, *, #187, .F. ) ;
#39539=DIRECTION ( 'NONE',  ( -0.000000000000000000, -0.000000000000000000, -1.000000000000000000 ) ) ;
#39561=EDGE_LOOP ( 'NONE', ( #1190, #22766, #45185, #28687 ) ) ;
#39569=EDGE_LOOP ( 'NONE', ( #13557, #39491, #9019, #45763 ) ) ;
#39573=CARTESIAN_POINT ( 'NONE',  ( -21.33958957442910886, -129.9559990355020034, 5.500000000000000000 ) ) ;
#39577=CARTESIAN_POINT ( 'NONE',  ( 1.474095553543393056, -119.7224350544041869, 2.500000000000000000 ) ) ;
#39583=VERTEX_POINT ( 'NONE', #32188 ) ;
#39635=SHAPE_REPRESENTATION_RELATIONSHIP ( 'NONE' , 'NONE' ,  #29385, #47339 ) ;
#39640=EDGE_CURVE ( 'NONE', #43899, #17111, #2791, .T. ) ;
#39657=DIRECTION ( 'NONE',  ( 0.9580045777625456616, 0.2867529058022021404, 0.000000000000000000 ) ) ;
#39673=EDGE_LOOP ( 'NONE', ( #2202, #45393, #45664, #26458 ) ) ;
#39680=DIRECTION ( 'NONE',  ( 0.2306669878475637314, 0.9730327541852493711, -0.000000000000000000 ) ) ;
#39699=EDGE_CURVE ( 'NONE', #16099, #19725, #29698, .T. ) ;
#39704=EDGE_LOOP ( 'NONE', ( #28671, #7242, #47736, #13431 ) ) ;
#39711=AXIS2_PLACEMENT_3D ( 'NONE', #41600, #8057, #30353 ) ;
#39715=FACE_OUTER_BOUND ( 'NONE', #45159, .T. ) ;
#39717=PLANE ( 'NONE',  #16569 ) ;
#39725=VERTEX_POINT ( 'NONE', #41217 ) ;
#39753=DIRECTION ( 'NONE',  ( 0.1276937514489679681, 0.9918136447140103451, 0.000000000000000000 ) ) ;
#39755=CARTESIAN_POINT ( 'NONE',  ( -0.8815729230226008184, -93.47222532549339746, 2.500000000000000000 ) ) ;
#39761=ORIENTED_EDGE ( 'NONE', *, *, #36433, .F. ) ;
#39782=DIRECTION ( 'NONE',  ( 0.4279312458753000703, 0.9038112904824842087, -0.000000000000000000 ) ) ;
#39799=VECTOR ( 'NONE', #4255, 1000.000000000000000 ) ;
#39800=EDGE_CURVE ( 'NONE', #5216, #23160, #1542, .T. ) ;
#39814=CARTESIAN_POINT ( 'NONE',  ( 21.85433023846371370, -135.0628101570779620, 5.500000000000000000 ) ) ;
#39825=VERTEX_POINT ( 'NONE', #23560 ) ;
#39845=LINE ( 'NONE', #10942, #31165 ) ;
#39864=ORIENTED_EDGE ( 'NONE', *, *, #34557, .T. ) ;
#39873=ORIENTED_EDGE ( 'NONE', *, *, #27187, .T. ) ;
#39886=CARTESIAN_POINT ( 'NONE',  ( 16.84844760790522855, -103.5491698323862124, 2.500000000000000000 ) ) ;
#39894=ORIENTED_EDGE ( 'NONE', *, *, #1090, .T. ) ;
#39905=ORIENTED_EDGE ( 'NONE', *, *, #6812, .F. ) ;
#39914=LINE ( 'NONE', #36228, #44117 ) ;
#39915=DIRECTION ( 'NONE',  ( -0.000000000000000000, -0.000000000000000000, -1.000000000000000000 ) ) ;
#39916=CARTESIAN_POINT ( 'NONE',  ( 0.000000000000000000, -120.0000000000000000, 2.500000000000000000 ) ) ;
#39923=VECTOR ( 'NONE', #14008, 1000.000000000000000 ) ;
#39940=CARTESIAN_POINT ( 'NONE',  ( -48.80839716909612491, -10.37454508288793065, -5.500000000000000000 ) ) ;
#39968=DIRECTION ( 'NONE',  ( -0.4279312458752990711, -0.9038112904824846527, 0.000000000000000000 ) ) ;
#39969=EDGE_CURVE ( 'NONE', #28791, #41996, #722, .T. ) ;
#39973=EDGE_CURVE ( 'NONE', #18975, #3694, #12024, .T. ) ;
#39982=ADVANCED_FACE ( 'NONE', ( #7594 ), #34484, .T. ) ;
#39988=LINE ( 'NONE', #14030, #40961 ) ;
#40001=PLANE ( 'NONE',  #32800 ) ;
#40004=EDGE_CURVE ( 'NONE', #17292, #6288, #494, .T. ) ;
#40020=LINE ( 'NONE', #13842, #16718 ) ;
#40037=ADVANCED_FACE ( 'NONE', ( #43182 ), #46859, .F. ) ;
#40046=ORIENTED_EDGE ( 'NONE', *, *, #3914, .T. ) ;
#40056=EDGE_CURVE ( 'NONE', #30905, #28317, #28022, .T. ) ;
#40068=VERTEX_POINT ( 'NONE', #38806 ) ;
#40079=PRESENTATION_STYLE_ASSIGNMENT (( #28814 ) ) ;
#40084=ORIENTED_EDGE ( 'NONE', *, *, #7125, .F. ) ;
#40086=FACE_OUTER_BOUND ( 'NONE', #47001, .T. ) ;
#40087=VECTOR ( 'NONE', #44133, 1000.000000000000114 ) ;
#40089=CARTESIAN_POINT ( 'NONE',  ( 22.94323693612312809, -114.6983135802921083, 5.500000000000000000 ) ) ;
#40094=EDGE_LOOP ( 'NONE', ( #32277, #1785, #33862, #13946 ) ) ;
#40109=LINE ( 'NONE', #6570, #26131 ) ;
#40125=ADVANCED_FACE ( 'NONE', ( #5495 ), #21634, .T. ) ;
#40133=DIRECTION ( 'NONE',  ( -0.08130631524010117905, 0.9966891607226784355, 0.000000000000000000 ) ) ;
#40140=EDGE_LOOP ( 'NONE', ( #35170, #23827, #28364, #4016 ) ) ;
#40142=DIRECTION ( 'NONE',  ( 0.000000000000000000, 0.000000000000000000, 1.000000000000000000 ) ) ;
#40144=ORIENTED_EDGE ( 'NONE', *, *, #8189, .F. ) ;
#40148=DIRECTION ( 'NONE',  ( 0.5687579148473744795, -0.8225049752423790883, 0.000000000000000000 ) ) ;
#40185=FACE_OUTER_BOUND ( 'NONE', #15458, .T. ) ;
#40191=DIRECTION ( 'NONE',  ( 0.6691306063588569053, 0.7431448254773954654, 0.000000000000000000 ) ) ;
#40193=CARTESIAN_POINT ( 'NONE',  ( 21.07894319797337346, -103.8699611390234878, 2.500000000000000000 ) ) ;
#40206=LINE ( 'NONE', #40924, #11265 ) ;
#40208=DIRECTION ( 'NONE',  ( -0.08130631524009862554, 0.9966891607226787686, 0.000000000000000000 ) ) ;
#40209=EDGE_LOOP ( 'NONE', ( #27500, #669, #44400, #8235 ) ) ;
#40211=PRODUCT ( 'Sliding Dog Clutch Collar', 'Sliding Dog Clutch Collar', '', ( #46303 ) ) ;
#40213=CARTESIAN_POINT ( 'NONE',  ( -0.7800914985199643992, -121.2811936832255100, 2.500000000000000000 ) ) ;
#40223=DIRECTION ( 'NONE',  ( -0.6064928550163533050, -0.7950889364178781449, 0.000000000000000000 ) ) ;
#40229=CARTESIAN_POINT ( 'NONE',  ( -10.21100092698785033, -95.54625877152835756, 2.500000000000000000 ) ) ;
#40242=EDGE_CURVE ( 'NONE', #18493, #41154, #2527, .T. ) ;
#40271=FACE_OUTER_BOUND ( 'NONE', #20792, .T. ) ;
#40274=PLANE ( 'NONE',  #43175 ) ;
#40298=EDGE_LOOP ( 'NONE', ( #25730, #44512, #34981, #6820 ) ) ;
#40311=DIRECTION ( 'NONE',  ( -0.5687579148473752566, 0.8225049752423786442, 0.000000000000000000 ) ) ;
#40330=FACE_BOUND ( 'NONE', #4398, .T. ) ;
#40334=VECTOR ( 'NONE', #16955, 1000.000000000000000 ) ;
#40336=LINE ( 'NONE', #18268, #22730 ) ;
#40357=ORIENTED_EDGE ( 'NONE', *, *, #12757, .F. ) ;
#40358=AXIS2_PLACEMENT_3D ( 'NONE', #14255, #29175, #44114 ) ;
#40366=EDGE_LOOP ( 'NONE', ( #20194, #36013, #6069, #24981 ) ) ;
#40401=ADVANCED_FACE ( 'NONE', ( #30659 ), #45579, .F. ) ;
#40407=ORIENTED_EDGE ( 'NONE', *, *, #13322, .F. ) ;
#40411=FACE_OUTER_BOUND ( 'NONE', #31727, .T. ) ;
#40426=VECTOR ( 'NONE', #2058, 1000.000000000000000 ) ;
#40430=ORIENTED_EDGE ( 'NONE', *, *, #38501, .T. ) ;
#40434=CARTESIAN_POINT ( 'NONE',  ( 0.7800914985199594032, -118.7188063167744900, -2.500000000000000000 ) ) ;
#40437=CARTESIAN_POINT ( 'NONE',  ( 12.13205353604972991, -140.1820037904669789, 5.500000000000000000 ) ) ;
#40444=DIRECTION ( 'NONE',  ( -0.000000000000000000, -0.000000000000000000, -1.000000000000000000 ) ) ;
#40452=CARTESIAN_POINT ( 'NONE',  ( 18.80329974962065265, -105.8248132807389084, 5.500000000000000000 ) ) ;
#40458=LINE ( 'NONE', #21109, #9154 ) ;
#40459=LINE ( 'NONE', #2994, #45041 ) ;
#40485=DIRECTION ( 'NONE',  ( 0.9227826878668550226, 0.3853207896976523772, -0.000000000000000000 ) ) ;
#40487=VECTOR ( 'NONE', #8965, 1000.000000000000000 ) ;
#40506=VECTOR ( 'NONE', #26586, 1000.000000000000114 ) ;
#40510=LINE ( 'NONE', #7207, #44316 ) ;
#40512=PLANE ( 'NONE',  #173 ) ;
#40526=ORIENTED_EDGE ( 'NONE', *, *, #43982, .T. ) ;
#40534=DIRECTION ( 'NONE',  ( -0.1045284632676436315, -0.9945218953682742891, 0.000000000000000000 ) ) ;
#40535=ORIENTED_EDGE ( 'NONE', *, *, #28354, .F. ) ;
#40536=CARTESIAN_POINT ( 'NONE',  ( 23.49916127795269460, -121.5130826919798039, 5.500000000000000000 ) ) ;
#40540=CARTESIAN_POINT ( 'NONE',  ( 22.94323693612312809, -114.6983135802921083, -5.500000000000000000 ) ) ;
#40542=FACE_BOUND ( 'NONE', #18773, .T. ) ;
#40548=CARTESIAN_POINT ( 'NONE',  ( 14.59956846177685996, -138.4757300459248484, -5.500000000000000000 ) ) ;
#40549=EDGE_CURVE ( 'NONE', #20931, #10647, #38981, .T. ) ;
#40559=CARTESIAN_POINT ( 'NONE',  ( 5.822613034544236399, -142.8165987265839760, 5.500000000000000000 ) ) ;
#40568=CYLINDRICAL_SURFACE ( 'NONE', #13813, 30.50000000000000000 ) ;
#40577=ORIENTED_EDGE ( 'NONE', *, *, #28247, .F. ) ;
#40578=AXIS2_PLACEMENT_3D ( 'NONE', #3369, #18306, #33245 ) ;
#40599=EDGE_CURVE ( 'NONE', #17612, #41379, #10800, .T. ) ;
#40627=CARTESIAN_POINT ( 'NONE',  ( -32.50000000000000000, -120.0000000000000000, 2.500000000000000000 ) ) ;
#40654=DIRECTION ( 'NONE',  ( 1.000000000000000000, 0.000000000000000000, 0.000000000000000000 ) ) ;
#40660=EDGE_LOOP ( 'NONE', ( #39385, #8974, #24715, #13549 ) ) ;
#40667=EDGE_LOOP ( 'NONE', ( #14840, #19344, #37179, #3082 ) ) ;
#40673=DIRECTION ( 'NONE',  ( -0.7950889364178781449, 0.6064928550163533050, 0.000000000000000000 ) ) ;
#40684=DIRECTION ( 'NONE',  ( -0.6516173805718079581, 0.7585478161175706058, 0.000000000000000000 ) ) ;
#40694=ORIENTED_EDGE ( 'NONE', *, *, #42773, .F. ) ;
#40712=VERTEX_POINT ( 'NONE', #730 ) ;
#40720=AXIS2_PLACEMENT_3D ( 'NONE', #24959, #2213, #17137 ) ;
#40734=EDGE_LOOP ( 'NONE', ( #3365, #5588, #15623, #24330 ) ) ;
#40738=CARTESIAN_POINT ( 'NONE',  ( -1.474095553543409487, -120.2775649455957989, 2.500000000000000000 ) ) ;
#40757=VECTOR ( 'NONE', #23634, 1000.000000000000000 ) ;
#40770=ADVANCED_FACE ( 'NONE', ( #509 ), #33309, .T. ) ;
#40772=CARTESIAN_POINT ( 'NONE',  ( 119.3426274441929280, -132.5434155921172419, 5.500000000000000000 ) ) ;
#40783=ORIENTED_EDGE ( 'NONE', *, *, #42660, .F. ) ;
#40790=CARTESIAN_POINT ( 'NONE',  ( -26.29030328629083968, -123.6496510949466341, -5.500000000000000000 ) ) ;
#40799=CARTESIAN_POINT ( 'NONE',  ( -23.97194136764370498, -131.3950000906648938, 5.500000000000000000 ) ) ;
#40829=CARTESIAN_POINT ( 'NONE',  ( -0.9774260708577104939, -118.8621782758236378, -2.500000000000000000 ) ) ;
#40838=DIRECTION ( 'NONE',  ( -0.9227826878668540234, -0.3853207896976546531, 0.000000000000000000 ) ) ;
#40846=VERTEX_POINT ( 'NONE', #15918 ) ;
#40854=PLANE ( 'NONE',  #22879 ) ;
#40858=CARTESIAN_POINT ( 'NONE',  ( -19.90058851926621841, -132.5883508287165853, -2.500000000000000000 ) ) ;
#40866=DIRECTION ( 'NONE',  ( 0.9580045777625452175, 0.2867529058022035837, -0.000000000000000000 ) ) ;
#40890=CARTESIAN_POINT ( 'NONE',  ( 23.11608002360578240, -124.4885236261218182, 5.500000000000000000 ) ) ;
#40900=DIRECTION ( 'NONE',  ( 0.000000000000000000, -0.000000000000000000, -1.000000000000000000 ) ) ;
#40924=CARTESIAN_POINT ( 'NONE',  ( -6.880223345695647197, -142.5202692415819854, 5.500000000000000000 ) ) ;
#40936=AXIS2_PLACEMENT_3D ( 'NONE', #17964, #3041, #13585 ) ;
#40946=VECTOR ( 'NONE', #36352, 1000.000000000000114 ) ;
#40958=VERTEX_POINT ( 'NONE', #13213 ) ;
#40961=VECTOR ( 'NONE', #48039, 1000.000000000000000 ) ;
#40968=VECTOR ( 'NONE', #46397, 1000.000000000000114 ) ;
#40969=CARTESIAN_POINT ( 'NONE',  ( -21.33958957442910886, -129.9559990355020034, 5.500000000000000000 ) ) ;
#40979=VECTOR ( 'NONE', #41307, 1000.000000000000114 ) ;
#40989=CARTESIAN_POINT ( 'NONE',  ( 26.47460221209471598, -121.8961639463267090, 2.500000000000000000 ) ) ;
#40999=DIRECTION ( 'NONE',  ( 0.8225049752423776450, 0.5687579148473764779, 0.000000000000000000 ) ) ;
#41004=AXIS2_PLACEMENT_3D ( 'NONE', #44527, #32776, #25189 ) ;
#41011=EDGE_CURVE ( 'NONE', #19725, #16756, #30858, .T. ) ;
#41017=EDGE_LOOP ( 'NONE', ( #474, #32267, #21990, #25555 ) ) ;
#41032=DIRECTION ( 'NONE',  ( 0.7950889364178788110, -0.6064928550163524168, 0.000000000000000000 ) ) ;
#41035=ORIENTED_EDGE ( 'NONE', *, *, #6251, .F. ) ;
#41038=DIRECTION ( 'NONE',  ( -0.4796670183876317051, 0.8774505977381971134, 0.000000000000000000 ) ) ;
#41042=FACE_BOUND ( 'NONE', #23330, .T. ) ;
#41051=DIRECTION ( 'NONE',  ( 0.9435911131814398445, -0.3311129884571295534, 0.000000000000000000 ) ) ;
#41071=FACE_OUTER_BOUND ( 'NONE', #37155, .T. ) ;
#41078=DIRECTION ( 'NONE',  ( 0.7273375899149802093, -0.6862798483830544471, 0.000000000000000000 ) ) ;
#41082=EDGE_CURVE ( 'NONE', #41996, #44807, #3130, .T. ) ;
#41085=FACE_OUTER_BOUND ( 'NONE', #1897, .T. ) ;
#41086=LINE ( 'NONE', #37394, #17520 ) ;
#41108=ORIENTED_EDGE ( 'NONE', *, *, #17642, .T. ) ;
#41121=CARTESIAN_POINT ( 'NONE',  ( -25.00516449930816876, -111.2255058058861010, 2.500000000000000000 ) ) ;
#41122=EDGE_CURVE ( 'NONE', #46691, #21034, #13694, .T. ) ;
#41128=CARTESIAN_POINT ( 'NONE',  ( 12.69589495141918611, -96.69089767102708777, 5.500000000000000000 ) ) ;
#41135=FACE_OUTER_BOUND ( 'NONE', #14361, .T. ) ;
#41143=VECTOR ( 'NONE', #6858, 999.9999999999998863 ) ;
#41153=EDGE_LOOP ( 'NONE', ( #6938, #2285, #3803, #30728 ) ) ;
#41154=VERTEX_POINT ( 'NONE', #43554 ) ;
#41155=ORIENTED_EDGE ( 'NONE', *, *, #38416, .T. ) ;
#41164=LINE ( 'NONE', #3700, #16918 ) ;
#41169=DIRECTION ( 'NONE',  ( 1.000000000000000000, 0.000000000000000000, 0.000000000000000000 ) ) ;
#41172=CARTESIAN_POINT ( 'NONE',  ( -0.9515373497862389396, -96.47140937769621871, -5.500000000000000000 ) ) ;
#41175=PLANE ( 'NONE',  #5178 ) ;
#41184=CARTESIAN_POINT ( 'NONE',  ( 11.34017801569539685, -96.04900080221412395, 2.500000000000000000 ) ) ;
#41196=ADVANCED_FACE ( 'NONE', ( #30070 ), #14660, .F. ) ;
#41208=ORIENTED_EDGE ( 'NONE', *, *, #21048, .F. ) ;
#41209=AXIS2_PLACEMENT_3D ( 'NONE', #6031, #35638, #17026 ) ;
#41217=CARTESIAN_POINT ( 'NONE',  ( 21.07894319797337701, -103.8699611390234878, 5.500000000000000000 ) ) ;
#41218=AXIS2_PLACEMENT_3D ( 'NONE', #21395, #28979, #21646 ) ;
#41221=EDGE_CURVE ( 'NONE', #8139, #13979, #26401, .T. ) ;
#41238=CARTESIAN_POINT ( 'NONE',  ( -19.90058851926621131, -132.5883508287165853, 5.500000000000000000 ) ) ;
#41239=VECTOR ( 'NONE', #27695, 1000.000000000000227 ) ;
#41259=VERTEX_POINT ( 'NONE', #22955 ) ;
#41264=VERTEX_POINT ( 'NONE', #10975 ) ;
#41266=DIRECTION ( 'NONE',  ( 0.6064928550163524168, 0.7950889364178788110, 0.000000000000000000 ) ) ;
#41294=DIRECTION ( 'NONE',  ( 0.1850432970638682395, -0.9827303690289279636, 0.000000000000000000 ) ) ;
#41300=CARTESIAN_POINT ( 'NONE',  ( -32.50000000000000000, -120.0000000000000000, 2.500000000000000000 ) ) ;
#41301=DIRECTION ( 'NONE',  ( 0.1276937514489679681, 0.9918136447140103451, 0.000000000000000000 ) ) ;
#41303=EDGE_CURVE ( 'NONE', #7858, #41627, #19033, .T. ) ;
#41305=FACE_OUTER_BOUND ( 'NONE', #13612, .T. ) ;
#41307=DIRECTION ( 'NONE',  ( 0.6516173805718079581, -0.7585478161175704948, 0.000000000000000000 ) ) ;
#41309=FACE_OUTER_BOUND ( 'NONE', #40209, .T. ) ;
#41317=PLANE ( 'NONE',  #17888 ) ;
#41332=ORIENTED_EDGE ( 'NONE', *, *, #28126, .T. ) ;
#41336=ADVANCED_FACE ( 'NONE', ( #34939 ), #27601, .F. ) ;
#41344=VERTEX_POINT ( 'NONE', #20006 ) ;
#41345=STYLED_ITEM ( 'NONE', ( #17320 ), #47339 ) ;
#41354=DIRECTION ( 'NONE',  ( 0.8225049752423786442, 0.5687579148473752566, -0.000000000000000000 ) ) ;
#41360=CARTESIAN_POINT ( 'NONE',  ( -20.30386590532152979, -102.9045904027214959, 5.500000000000000000 ) ) ;
#41379=VERTEX_POINT ( 'NONE', #38374 ) ;
#41385=ORIENTED_EDGE ( 'NONE', *, *, #11007, .F. ) ;
#41405=LINE ( 'NONE', #30879, #39319 ) ;
#41417=FACE_BOUND ( 'NONE', #24280, .T. ) ;
#41442=ORIENTED_EDGE ( 'NONE', *, *, #8538, .T. ) ;
#41454=ORIENTED_EDGE ( 'NONE', *, *, #16091, .F. ) ;
#41463=LINE ( 'NONE', #22382, #13368 ) ;
#41468=DIRECTION ( 'NONE',  ( 0.2867529058022035837, -0.9580045777625452175, 0.000000000000000000 ) ) ;
#41472=VECTOR ( 'NONE', #24475, 1000.000000000000000 ) ;
#41475=LINE ( 'NONE', #11131, #45110 ) ;
#41486=ADVANCED_FACE ( 'NONE', ( #9961 ), #10441, .F. ) ;
#41499=DIRECTION ( 'NONE',  ( -0.000000000000000000, -0.000000000000000000, -1.000000000000000000 ) ) ;
#41519=PLANE ( 'NONE',  #25258 ) ;
#41524=CARTESIAN_POINT ( 'NONE',  ( -15.44521549751111422, -137.7748507232956001, -5.500000000000000000 ) ) ;
#41533=VECTOR ( 'NONE', #40133, 1000.000000000000227 ) ;
#41537=CARTESIAN_POINT ( 'NONE',  ( 26.09152095774781799, -124.8716048804687375, -5.500000000000000000 ) ) ;
#41544=DIRECTION ( 'NONE',  ( -0.9730327541852497042, 0.2306669878475623159, 0.000000000000000000 ) ) ;
#41551=FACE_OUTER_BOUND ( 'NONE', #10461, .T. ) ;
#41563=VECTOR ( 'NONE', #24417, 1000.000000000000000 ) ;
#41568=ORIENTED_EDGE ( 'NONE', *, *, #6156, .F. ) ;
#41575=DIRECTION ( 'NONE',  ( 1.000000000000000000, 0.000000000000000000, 0.000000000000000000 ) ) ;
#41600=CARTESIAN_POINT ( 'NONE',  ( -26.53422223201112828, -120.6595836127786043, 5.500000000000000000 ) ) ;
#41620=EDGE_CURVE ( 'NONE', #33189, #43507, #18971, .T. ) ;
#41627=VERTEX_POINT ( 'NONE', #29528 ) ;
#41630=PLANE ( 'NONE',  #22696 ) ;
#41643=PLANE ( 'NONE',  #46184 ) ;
#41660=ADVANCED_FACE ( 'NONE', ( #40542, #36856, #44688, #3324, #11168, #18256, #26093, #41042, #37351, #13278, #24776, #9121, #35060, #5221, #31412, #32127, #16235 ), #42411, .T. ) ;
#41669=ADVANCED_FACE ( 'NONE', ( #28198 ), #39717, .F. ) ;
#41673=EDGE_CURVE ( 'NONE', #34735, #19426, #27977, .T. ) ;
#41691=CARTESIAN_POINT ( 'NONE',  ( 11.41210121379328335, -99.40233154247455616, 5.500000000000000000 ) ) ;
#41700=DIRECTION ( 'NONE',  ( 0.7273375899149802093, -0.6862798483830544471, 0.000000000000000000 ) ) ;
#41711=LINE ( 'NONE', #42433, #30134 ) ;
#41719=CARTESIAN_POINT ( 'NONE',  ( 21.85433023846371370, -135.0628101570779620, -5.500000000000000000 ) ) ;
#41732=ADVANCED_FACE ( 'NONE', ( #46086 ), #20360, .F. ) ;
#41733=VERTEX_POINT ( 'NONE', #46576 ) ;
#41739=ORIENTED_EDGE ( 'NONE', *, *, #47671, .F. ) ;
#41742=CARTESIAN_POINT ( 'NONE',  ( -8.826826895187510402, -94.96827758698185562, 5.500000000000000000 ) ) ;
#41764=LINE ( 'NONE', #44703, #35438 ) ;
#41769=CARTESIAN_POINT ( 'NONE',  ( 19.12409105625795291, -101.5943176906707919, 5.500000000000000000 ) ) ;
#41792=EDGE_CURVE ( 'NONE', #14101, #16743, #44333, .T. ) ;
#41798=ADVANCED_FACE ( 'NONE', ( #36260 ), #48246, .F. ) ;
#41803=FACE_OUTER_BOUND ( 'NONE', #17666, .T. ) ;
#41815=VECTOR ( 'NONE', #66, 1000.000000000000000 ) ;
#41819=ORIENTED_EDGE ( 'NONE', *, *, #22803, .F. ) ;
#41879=ORIENTED_EDGE ( 'NONE', *, *, #15155, .T. ) ;
#41880=LINE ( 'NONE', #8332, #28255 ) ;
#41891=CARTESIAN_POINT ( 'NONE',  ( 2.117611129180199558, -93.54218975225703048, 5.500000000000000000 ) ) ;
#41900=CARTESIAN_POINT ( 'NONE',  ( -26.53422223201112828, -120.6595836127786043, 5.500000000000000000 ) ) ;
#41912=DIRECTION ( 'NONE',  ( 0.000000000000000000, 0.000000000000000000, -1.000000000000000000 ) ) ;
#41933=DIRECTION ( 'NONE',  ( -0.7585478161175716050, -0.6516173805718067369, 0.000000000000000000 ) ) ;
#41936=EDGE_CURVE ( 'NONE', #42659, #28062, #4664, .T. ) ;
#41940=VERTEX_POINT ( 'NONE', #11536 ) ;
#41947=VERTEX_POINT ( 'NONE', #8090 ) ;
#41950=ORIENTED_EDGE ( 'NONE', *, *, #36423, .T. ) ;
#41958=CARTESIAN_POINT ( 'NONE',  ( -3.961125083139900749, -143.2122702051246677, 2.500000000000000000 ) ) ;
#41964=PLANE ( 'NONE',  #11940 ) ;
#41980=VECTOR ( 'NONE', #7757, 1000.000000000000000 ) ;
#41996=VERTEX_POINT ( 'NONE', #3942 ) ;
#42012=LINE ( 'NONE', #38328, #285 ) ;
#42016=CARTESIAN_POINT ( 'NONE',  ( 20.85212586905262100, -130.9402397935870965, 5.500000000000000000 ) ) ;
#42026=DIRECTION ( 'NONE',  ( 0.7273375899149793211, -0.6862798483830554463, 0.000000000000000000 ) ) ;
#42037=VECTOR ( 'NONE', #35266, 1000.000000000000000 ) ;
#42041=VECTOR ( 'NONE', #25201, 1000.000000000000000 ) ;
#42055=CARTESIAN_POINT ( 'NONE',  ( 20.85212586905262100, -130.9402397935870965, -5.500000000000000000 ) ) ;
#42058=CARTESIAN_POINT ( 'NONE',  ( 9.984461079971730157, -95.40710393340120277, 5.500000000000000000 ) ) ;
#42065=ORIENTED_EDGE ( 'NONE', *, *, #3950, .T. ) ;
#42066=EDGE_CURVE ( 'NONE', #39318, #31838, #44812, .T. ) ;
#42081=CARTESIAN_POINT ( 'NONE',  ( -4.653126046682595884, -146.1313684676804314, 5.500000000000000000 ) ) ;
#42085=( NAMED_UNIT ( * ) SI_UNIT ( $, .STERADIAN. ) SOLID_ANGLE_UNIT ( ) );
#42090=VECTOR ( 'NONE', #1176, 1000.000000000000114 ) ;
#42091=CARTESIAN_POINT ( 'NONE',  ( -103.9230484541323705, -180.0000000000004832, 5.500000000000000000 ) ) ;
#42092=DIRECTION ( 'NONE',  ( 0.9038112904824853189, -0.4279312458752977388, 0.000000000000000000 ) ) ;
#42101=VERTEX_POINT ( 'NONE', #35730 ) ;
#42105=DIRECTION ( 'NONE',  ( -0.000000000000000000, -0.000000000000000000, -1.000000000000000000 ) ) ;
#42111=DIRECTION ( 'NONE',  ( 0.4279312458752976833, 0.9038112904824853189, -0.000000000000000000 ) ) ;
#42135=CARTESIAN_POINT ( 'NONE',  ( -3.961125083139900749, -143.2122702051246677, 5.500000000000000000 ) ) ;
#42136=PLANE ( 'NONE',  #38779 ) ;
#42138=FACE_OUTER_BOUND ( 'NONE', #32400, .T. ) ;
#42144=PLANE ( 'NONE',  #35440 ) ;
#42172=EDGE_LOOP ( 'NONE', ( #40783, #16612, #20233, #45898 ) ) ;
#42185=CARTESIAN_POINT ( 'NONE',  ( 0.000000000000000000, -120.0000000000000000, 5.500000000000000888 ) ) ;
#42190=AXIS2_PLACEMENT_3D ( 'NONE', #24274, #24984, #4533 ) ;
#42199=DIRECTION ( 'NONE',  ( -0.4796670183876317051, 0.8774505977381971134, 0.000000000000000000 ) ) ;
#42203=ORIENTED_EDGE ( 'NONE', *, *, #18464, .F. ) ;
#42210=PLANE ( 'NONE',  #46494 ) ;
#42216=AXIS2_PLACEMENT_3D ( 'NONE', #5379, #13444, #46251 ) ;
#42218=CARTESIAN_POINT ( 'NONE',  ( 6.377742925735834234, -145.7647898336708181, -5.500000000000000000 ) ) ;
#42226=ORIENTED_EDGE ( 'NONE', *, *, #31629, .T. ) ;
#42271=VERTEX_POINT ( 'NONE', #39886 ) ;
#42286=ORIENTED_EDGE ( 'NONE', *, *, #23360, .T. ) ;
#42294=VECTOR ( 'NONE', #18064, 1000.000000000000000 ) ;
#42337=EDGE_LOOP ( 'NONE', ( #27173, #21452, #21912, #46965 ) ) ;
#42368=DIRECTION ( 'NONE',  ( 0.4279312458752976833, 0.9038112904824853189, -0.000000000000000000 ) ) ;
#42394=EDGE_CURVE ( 'NONE', #31838, #7679, #45243, .T. ) ;
#42397=ORIENTED_EDGE ( 'NONE', *, *, #2251, .T. ) ;
#42398=CARTESIAN_POINT ( 'NONE',  ( 0.9774260708577211521, -121.1378217241763622, -2.500000000000000000 ) ) ;
#42411=PLANE ( 'NONE',  #34518 ) ;
#42433=CARTESIAN_POINT ( 'NONE',  ( 10.05638427806949586, -98.76043467366159234, 2.500000000000000000 ) ) ;
#42460=FACE_OUTER_BOUND ( 'NONE', #40140, .T. ) ;
#42465=DIRECTION ( 'NONE',  ( 0.9730327541852493711, -0.2306669878475637314, 0.000000000000000000 ) ) ;
#42480=PLANE ( 'NONE',  #31112 ) ;
#42482=CARTESIAN_POINT ( 'NONE',  ( -14.87942725330654348, -141.9795960975983178, 2.500000000000000000 ) ) ;
#42500=CARTESIAN_POINT ( 'NONE',  ( 5.822613034544236399, -142.8165987265839760, 5.500000000000000000 ) ) ;
#42528=VERTEX_POINT ( 'NONE', #9478 ) ;
#42529=ORIENTED_EDGE ( 'NONE', *, *, #18169, .T. ) ;
#42533=CARTESIAN_POINT ( 'NONE',  ( -23.54415474984308787, -120.4156646670583086, -5.500000000000000000 ) ) ;
#42544=CARTESIAN_POINT ( 'NONE',  ( -22.53294031248082163, -134.0273518838794757, -5.500000000000000000 ) ) ;
#42590=VECTOR ( 'NONE', #41933, 1000.000000000000000 ) ;
#42600=ORIENTED_EDGE ( 'NONE', *, *, #28424, .T. ) ;
#42609=EDGE_CURVE ( 'NONE', #16641, #17111, #38642, .T. ) ;
#42624=CARTESIAN_POINT ( 'NONE',  ( 89.17737905728634473, -39.70432723693593857, -5.500000000000000000 ) ) ;
#42628=AXIS2_PLACEMENT_3D ( 'NONE', #11986, #35147, #16808 ) ;
#42654=DIRECTION ( 'NONE',  ( -0.000000000000000000, -0.000000000000000000, -1.000000000000000000 ) ) ;
#42659=VERTEX_POINT ( 'NONE', #35682 ) ;
#42660=EDGE_CURVE ( 'NONE', #30819, #40068, #20986, .T. ) ;
#42662=VECTOR ( 'NONE', #29485, 1000.000000000000114 ) ;
#42685=LINE ( 'NONE', #15760, #61 ) ;
#42694=VERTEX_POINT ( 'NONE', #32253 ) ;
#42698=DIRECTION ( 'NONE',  ( -0.1850432970638656582, 0.9827303690289285187, 0.000000000000000000 ) ) ;
#42729=ORIENTED_EDGE ( 'NONE', *, *, #5477, .T. ) ;
#42731=AXIS2_PLACEMENT_3D ( 'NONE', #29842, #40866, #44774 ) ;
#42750=AXIS2_PLACEMENT_3D ( 'NONE', #4348, #11678, #15830 ) ;
#42762=VERTEX_POINT ( 'NONE', #26352 ) ;
#42764=AXIS2_PLACEMENT_3D ( 'NONE', #4789, #34628, #1110 ) ;
#42773=EDGE_CURVE ( 'NONE', #10102, #20850, #18745, .T. ) ;
#42796=EDGE_CURVE ( 'NONE', #41264, #30621, #41764, .T. ) ;
#42797=CARTESIAN_POINT ( 'NONE',  ( -11.59517495878806947, -96.12423995607481686, -5.500000000000000000 ) ) ;
#42814=VECTOR ( 'NONE', #27215, 1000.000000000000000 ) ;
#42823=DIRECTION ( 'NONE',  ( 0.9997280174009349762, -0.02332147558787671729, 0.000000000000000000 ) ) ;
#42824=DIRECTION ( 'NONE',  ( -0.9435911131814395114, 0.3311129884571304971, 0.000000000000000000 ) ) ;
#42836=EDGE_CURVE ( 'NONE', #30446, #4822, #22441, .T. ) ;
#42837=ORIENTED_EDGE ( 'NONE', *, *, #40056, .F. ) ;
#42847=ORIENTED_EDGE ( 'NONE', *, *, #44657, .F. ) ;
#42848=AXIS2_PLACEMENT_3D ( 'NONE', #36626, #14850, #25608 ) ;
#42854=LINE ( 'NONE', #1985, #35397 ) ;
#42855=CARTESIAN_POINT ( 'NONE',  ( -17.26469406256017791, -140.1601175325492648, 5.500000000000000000 ) ) ;
#42869=VECTOR ( 'NONE', #12931, 1000.000000000000000 ) ;
#42882=PLANE ( 'NONE',  #46394 ) ;
#42893=EDGE_CURVE ( 'NONE', #40712, #33189, #9192, .T. ) ;
#42896=LINE ( 'NONE', #8864, #5906 ) ;
#42923=DIRECTION ( 'NONE',  ( 1.000000000000000000, 0.000000000000000000, 0.000000000000000000 ) ) ;
#42924=LINE ( 'NONE', #35323, #39509 ) ;
#42937=LINE ( 'NONE', #28238, #37758 ) ;
#42949=DIRECTION ( 'NONE',  ( -0.9966891607226786576, -0.08130631524009861166, 0.000000000000000000 ) ) ;
#42953=DIRECTION ( 'NONE',  ( -0.000000000000000000, -0.000000000000000000, -1.000000000000000000 ) ) ;
#42964=LINE ( 'NONE', #12866, #29444 ) ;
#42989=CARTESIAN_POINT ( 'NONE',  ( 25.38712131070745315, -112.4010479962415872, -2.500000000000000000 ) ) ;
#42992=EDGE_CURVE ( 'NONE', #41344, #19426, #866, .T. ) ;
#42993=ORIENTED_EDGE ( 'NONE', *, *, #33686, .F. ) ;
#42996=EDGE_LOOP ( 'NONE', ( #46499, #35003, #29257, #24645 ) ) ;
#43005=EDGE_CURVE ( 'NONE', #1874, #14593, #42012, .T. ) ;
#43013=LINE ( 'NONE', #1648, #24098 ) ;
#43017=DIRECTION ( 'NONE',  ( 0.9227826878668550226, 0.3853207896976523772, -0.000000000000000000 ) ) ;
#43032=ORIENTED_EDGE ( 'NONE', *, *, #44548, .T. ) ;
#43038=PLANE ( 'NONE',  #44297 ) ;
#43039=DIRECTION ( 'NONE',  ( 1.000000000000000000, 0.000000000000000000, 0.000000000000000000 ) ) ;
#43051=EDGE_CURVE ( 'NONE', #25561, #29936, #40020, .T. ) ;
#43060=VECTOR ( 'NONE', #18009, 999.9999999999998863 ) ;
#43081=DIRECTION ( 'NONE',  ( 0.9997280174009349762, -0.02332147558787674158, 0.000000000000000000 ) ) ;
#43092=CARTESIAN_POINT ( 'NONE',  ( 12.50000000000000000, -107.5000000000000000, 2.500000000000000000 ) ) ;
#43093=FACE_OUTER_BOUND ( 'NONE', #29891, .T. ) ;
#43094=DIRECTION ( 'NONE',  ( -0.000000000000000000, -0.000000000000000000, -1.000000000000000000 ) ) ;
#43102=PLANE ( 'NONE',  #47898 ) ;
#43104=ADVANCED_FACE ( 'NONE', ( #40271 ), #36577, .F. ) ;
#43112=CARTESIAN_POINT ( 'NONE',  ( -35.50000000000000711, -120.0000000000000000, -2.500000000000000000 ) ) ;
#43117=ORIENTED_EDGE ( 'NONE', *, *, #160, .T. ) ;
#43136=ORIENTED_EDGE ( 'NONE', *, *, #10552, .F. ) ;
#43145=ORIENTED_EDGE ( 'NONE', *, *, #17987, .T. ) ;
#43147=ORIENTED_EDGE ( 'NONE', *, *, #33705, .T. ) ;
#43155=CARTESIAN_POINT ( 'NONE',  ( -15.44521549751111422, -137.7748507232956001, 5.500000000000000000 ) ) ;
#43168=ADVANCED_FACE ( 'NONE', ( #11607 ), #10648, .F. ) ;
#43175=AXIS2_PLACEMENT_3D ( 'NONE', #6732, #25559, #44415 ) ;
#43182=FACE_OUTER_BOUND ( 'NONE', #30200, .T. ) ;
#43191=DIRECTION ( 'NONE',  ( -0.9580045777625456616, -0.2867529058022021404, 0.000000000000000000 ) ) ;
#43193=VECTOR ( 'NONE', #40223, 1000.000000000000114 ) ;
#43197=ORIENTED_EDGE ( 'NONE', *, *, #38911, .T. ) ;
#43208=LINE ( 'NONE', #9669, #44928 ) ;
#43220=CARTESIAN_POINT ( 'NONE',  ( 22.08297821871651934, -111.8242998470044540, 5.500000000000000000 ) ) ;
#43221=DIRECTION ( 'NONE',  ( 0.7950889364178796992, -0.6064928550163510845, 0.000000000000000000 ) ) ;
#43248=VERTEX_POINT ( 'NONE', #22128 ) ;
#43250=CARTESIAN_POINT ( 'NONE',  ( -22.67106064244953245, -113.6342314410295842, 5.500000000000000000 ) ) ;
#43290=DIRECTION ( 'NONE',  ( -0.000000000000000000, -0.000000000000000000, -1.000000000000000000 ) ) ;
#43295=FILL_AREA_STYLE ('',( #34473 ) ) ;
#43299=ORIENTED_EDGE ( 'NONE', *, *, #43439, .F. ) ;
#43305=VECTOR ( 'NONE', #44106, 1000.000000000000227 ) ;
#43308=VECTOR ( 'NONE', #41051, 1000.000000000000114 ) ;
#43327=ADVANCED_FACE ( 'NONE', ( #31186 ), #23103, .T. ) ;
#43333=DIRECTION ( 'NONE',  ( -0.000000000000000000, -0.000000000000000000, 1.000000000000000000 ) ) ;
#43340=CARTESIAN_POINT ( 'NONE',  ( 16.30584220631899228, -140.9432449716519784, 5.500000000000000000 ) ) ;
#43347=LINE ( 'NONE', #24023, #33265 ) ;
#43353=CARTESIAN_POINT ( 'NONE',  ( 11.41210121379328335, -99.40233154247455616, 5.500000000000000000 ) ) ;
#43357=EDGE_CURVE ( 'NONE', #3234, #40846, #8638, .T. ) ;
#43368=EDGE_LOOP ( 'NONE', ( #39154, #31082, #23661, #7189 ) ) ;
#43388=DIRECTION ( 'NONE',  ( -0.000000000000000000, -0.000000000000000000, -1.000000000000000000 ) ) ;
#43393=ORIENTED_EDGE ( 'NONE', *, *, #38645, .T. ) ;
#43418=EDGE_CURVE ( 'NONE', #35093, #42101, #35317, .T. ) ;
#43439=EDGE_CURVE ( 'NONE', #12057, #12729, #8171, .T. ) ;
#43455=ORIENTED_EDGE ( 'NONE', *, *, #9037, .T. ) ;
#43457=DIRECTION ( 'NONE',  ( -0.000000000000000000, -0.000000000000000000, -1.000000000000000000 ) ) ;
#43465=CARTESIAN_POINT ( 'NONE',  ( 25.81725066941077529, -113.8380548628854854, 5.500000000000000000 ) ) ;
#43482=LINE ( 'NONE', #39577, #15825 ) ;
#43487=VERTEX_POINT ( 'NONE', #32383 ) ;
#43488=DIRECTION ( 'NONE',  ( -0.5200609990132993854, -0.8541291221503275466, 0.000000000000000000 ) ) ;
#43507=VERTEX_POINT ( 'NONE', #10096 ) ;
#43520=VERTEX_POINT ( 'NONE', #40858 ) ;
#43524=VERTEX_POINT ( 'NONE', #43155 ) ;
#43526=EDGE_CURVE ( 'NONE', #42271, #11749, #7321, .T. ) ;
#43531=CARTESIAN_POINT ( 'NONE',  ( 2.874421927457452952, -143.3717286177755739, 5.500000000000000000 ) ) ;
#43532=CARTESIAN_POINT ( 'NONE',  ( 25.81725066941077529, -113.8380548628854854, 5.500000000000000000 ) ) ;
#43537=ORIENTED_EDGE ( 'NONE', *, *, #11412, .T. ) ;
#43539=ADVANCED_FACE ( 'NONE', ( #22261 ), #46595, .F. ) ;
#43553=AXIS2_PLACEMENT_3D ( 'NONE', #327, #45130, #38503 ) ;
#43554=CARTESIAN_POINT ( 'NONE',  ( 8.700667342345820288, -98.11853780484867116, 2.500000000000000000 ) ) ;
#43557=ORIENTED_EDGE ( 'NONE', *, *, #45655, .F. ) ;
#43571=CARTESIAN_POINT ( 'NONE',  ( -0.8815729230226008184, -93.47222532549339746, 5.500000000000000000 ) ) ;
#43576=DIRECTION ( 'NONE',  ( -0.4796670183876317051, 0.8774505977381971134, 0.000000000000000000 ) ) ;
#43584=DIRECTION ( 'NONE',  ( -0.000000000000000000, -0.000000000000000000, -1.000000000000000000 ) ) ;
#43603=FACE_OUTER_BOUND ( 'NONE', #39444, .T. ) ;
#43629=LINE ( 'NONE', #47533, #37579 ) ;
#43636=DIRECTION ( 'NONE',  ( -0.000000000000000000, -0.000000000000000000, 1.000000000000000000 ) ) ;
#43673=CARTESIAN_POINT ( 'NONE',  ( 22.94323693612312809, -114.6983135802921083, 5.500000000000000000 ) ) ;
#43678=CARTESIAN_POINT ( 'NONE',  ( -6.880223345695647197, -142.5202692415819854, -2.500000000000000000 ) ) ;
#43689=LINE ( 'NONE', #9670, #16575 ) ;
#43697=AXIS2_PLACEMENT_3D ( 'NONE', #47101, #14051, #21642 ) ;
#43720=AXIS2_PLACEMENT_3D ( 'NONE', #42624, #47006, #31612 ) ;
#43722=ADVANCED_FACE ( 'NONE', ( #39394 ), #44677, .F. ) ;
#43735=ORIENTED_EDGE ( 'NONE', *, *, #15923, .T. ) ;
#43736=ORIENTED_EDGE ( 'NONE', *, *, #16923, .F. ) ;
#43744=SURFACE_SIDE_STYLE ('',( #47419 ) ) ;
#43763=EDGE_CURVE ( 'NONE', #47615, #8515, #2839, .T. ) ;
#43796=CARTESIAN_POINT ( 'NONE',  ( -20.30386590532152979, -102.9045904027214959, 5.500000000000000000 ) ) ;
#43800=DIRECTION ( 'NONE',  ( 1.000000000000000000, 0.000000000000000000, -0.000000000000000000 ) ) ;
#43804=CARTESIAN_POINT ( 'NONE',  ( 18.80329974962065265, -105.8248132807389084, -5.500000000000000000 ) ) ;
#43806=PLANE ( 'NONE',  #39379 ) ;
#43811=EDGE_CURVE ( 'NONE', #25213, #22663, #29276, .T. ) ;
#43840=DIRECTION ( 'NONE',  ( 0.000000000000000000, -0.000000000000000000, 1.000000000000000000 ) ) ;
#43841=CARTESIAN_POINT ( 'NONE',  ( -22.53294031248081808, -134.0273518838794757, -2.500000000000000000 ) ) ;
#43847=DIRECTION ( 'NONE',  ( -0.4999999999999919509, -0.8660254037844432595, 0.000000000000000000 ) ) ;
#43863=EDGE_CURVE ( 'NONE', #9209, #29936, #8441, .T. ) ;
#43866=CARTESIAN_POINT ( 'NONE',  ( -17.09243336300205129, -103.8724235629982502, -2.500000000000000000 ) ) ;
#43874=VECTOR ( 'NONE', #38581, 1000.000000000000000 ) ;
#43886=VERTEX_POINT ( 'NONE', #34144 ) ;
#43899=VERTEX_POINT ( 'NONE', #122 ) ;
#43904=CARTESIAN_POINT ( 'NONE',  ( -11.59517495878806947, -96.12423995607481686, 5.500000000000000000 ) ) ;
#43912=ADVANCED_FACE ( 'NONE', ( #4536 ), #42210, .F. ) ;
#43920=CARTESIAN_POINT ( 'NONE',  ( 23.41451323550362318, -132.5004227906269989, -2.500000000000000000 ) ) ;
#43971=EDGE_LOOP ( 'NONE', ( #22892, #33850, #23531, #17200 ) ) ;
#43974=VERTEX_POINT ( 'NONE', #20933 ) ;
#43978=FACE_BOUND ( 'NONE', #24517, .T. ) ;
#43982=EDGE_CURVE ( 'NONE', #16743, #4190, #2318, .T. ) ;
#43996=DIRECTION ( 'NONE',  ( -0.9580045777625456616, -0.2867529058022021404, 0.000000000000000000 ) ) ;
#44001=EDGE_CURVE ( 'NONE', #30621, #30136, #13347, .T. ) ;
#44014=ORIENTED_EDGE ( 'NONE', *, *, #20898, .T. ) ;
#44017=VERTEX_POINT ( 'NONE', #47110 ) ;
#44021=ORIENTED_EDGE ( 'NONE', *, *, #10889, .F. ) ;
#44025=CARTESIAN_POINT ( 'NONE',  ( -1.233757462863590115, -120.8531368722710795, 2.500000000000000000 ) ) ;
#44053=CARTESIAN_POINT ( 'NONE',  ( -12.50000000000000000, -132.5000000000000000, 2.500000000000000000 ) ) ;
#44057=DIRECTION ( 'NONE',  ( 0.9227826878668540234, 0.3853207896976547087, -0.000000000000000000 ) ) ;
#44066=VECTOR ( 'NONE', #30747, 1000.000000000000114 ) ;
#44068=CARTESIAN_POINT ( 'NONE',  ( 21.07894319797337701, -103.8699611390234878, 5.500000000000000000 ) ) ;
#44078=ORIENTED_EDGE ( 'NONE', *, *, #1759, .F. ) ;
#44079=DIRECTION ( 'NONE',  ( -0.000000000000000000, -0.000000000000000000, 1.000000000000000000 ) ) ;
#44087=DIRECTION ( 'NONE',  ( -0.000000000000000000, -0.000000000000000000, 1.000000000000000000 ) ) ;
#44106=DIRECTION ( 'NONE',  ( 0.9966891607226786576, 0.08130631524009862554, 0.000000000000000000 ) ) ;
#44114=DIRECTION ( 'NONE',  ( 0.3090169943749448977, 0.9510565162951543083, 0.000000000000000000 ) ) ;
#44117=VECTOR ( 'NONE', #10533, 1000.000000000000000 ) ;
#44124=ORIENTED_EDGE ( 'NONE', *, *, #42066, .T. ) ;
#44131=DIRECTION ( 'NONE',  ( 0.000000000000000000, 0.000000000000000000, 1.000000000000000000 ) ) ;
#44132=ORIENTED_EDGE ( 'NONE', *, *, #3255, .T. ) ;
#44133=DIRECTION ( 'NONE',  ( 0.8225049752423776450, 0.5687579148473765889, -0.000000000000000000 ) ) ;
#44137=EDGE_CURVE ( 'NONE', #1537, #17280, #31697, .T. ) ;
#44142=ORIENTED_EDGE ( 'NONE', *, *, #45302, .F. ) ;
#44143=EDGE_CURVE ( 'NONE', #13979, #16986, #37304, .T. ) ;
#44144=AXIS2_PLACEMENT_3D ( 'NONE', #30252, #30984, #19936 ) ;
#44145=CIRCLE ( 'NONE', #23048, 30.50000000000000000 ) ;
#44148=VECTOR ( 'NONE', #39502, 999.9999999999998863 ) ;
#44194=ORIENTED_EDGE ( 'NONE', *, *, #1148, .T. ) ;
#44198=ORIENTED_EDGE ( 'NONE', *, *, #15266, .T. ) ;
#44209=ORIENTED_EDGE ( 'NONE', *, *, #4204, .T. ) ;
#44213=ORIENTED_EDGE ( 'NONE', *, *, #19375, .F. ) ;
#44217=DIRECTION ( 'NONE',  ( 0.9580045777625456616, 0.2867529058022021404, 0.000000000000000000 ) ) ;
#44228=FACE_OUTER_BOUND ( 'NONE', #35200, .T. ) ;
#44242=DIRECTION ( 'NONE',  ( 0.000000000000000000, 0.000000000000000000, 1.000000000000000000 ) ) ;
#44248=DIRECTION ( 'NONE',  ( 0.000000000000000000, 0.000000000000000000, 1.000000000000000000 ) ) ;
#44253=ORIENTED_EDGE ( 'NONE', *, *, #10552, .T. ) ;
#44261=ORIENTED_EDGE ( 'NONE', *, *, #1604, .F. ) ;
#44280=DIRECTION ( 'NONE',  ( 0.7585478161175716050, 0.6516173805718067369, 0.000000000000000000 ) ) ;
#44288=ORIENTED_EDGE ( 'NONE', *, *, #15088, .F. ) ;
#44289=ORIENTED_EDGE ( 'NONE', *, *, #16677, .F. ) ;
#44294=DIRECTION ( 'NONE',  ( -0.9580045777625456616, -0.2867529058022021404, 0.000000000000000000 ) ) ;
#44297=AXIS2_PLACEMENT_3D ( 'NONE', #35919, #9492, #39366 ) ;
#44304=LINE ( 'NONE', #40627, #38125 ) ;
#44314=ORIENTED_EDGE ( 'NONE', *, *, #6629, .F. ) ;
#44316=VECTOR ( 'NONE', #14076, 1000.000000000000000 ) ;
#44322=EDGE_LOOP ( 'NONE', ( #7108, #28154, #43145, #482 ) ) ;
#44333=LINE ( 'NONE', #6888, #33752 ) ;
#44337=AXIS2_PLACEMENT_3D ( 'NONE', #23118, #38054, #18706 ) ;
#44343=CARTESIAN_POINT ( 'NONE',  ( -23.54415474984308787, -120.4156646670583086, 5.500000000000000000 ) ) ;
#44351=CARTESIAN_POINT ( 'NONE',  ( -19.90058851926621131, -132.5883508287165853, -5.500000000000000000 ) ) ;
#44366=DIRECTION ( 'NONE',  ( 1.000000000000000000, 0.000000000000000000, 0.000000000000000000 ) ) ;
#44373=VECTOR ( 'NONE', #23767, 1000.000000000000000 ) ;
#44376=LINE ( 'NONE', #26500, #30716 ) ;
#44389=LINE ( 'NONE', #22106, #22280 ) ;
#44393=VECTOR ( 'NONE', #29032, 1000.000000000000000 ) ;
#44394=ORIENTED_EDGE ( 'NONE', *, *, #11718, .F. ) ;
#44400=ORIENTED_EDGE ( 'NONE', *, *, #38543, .T. ) ;
#44413=DIRECTION ( 'NONE',  ( 0.4796670183876317051, -0.8774505977381972244, 0.000000000000000000 ) ) ;
#44415=DIRECTION ( 'NONE',  ( -0.8225049752423776450, -0.5687579148473765889, 0.000000000000000000 ) ) ;
#44442=VERTEX_POINT ( 'NONE', #46334 ) ;
#44444=FACE_OUTER_BOUND ( 'NONE', #21313, .T. ) ;
#44454=ORIENTED_EDGE ( 'NONE', *, *, #8404, .F. ) ;
#44463=CARTESIAN_POINT ( 'NONE',  ( -9.055038557894883766, -98.31460683512894150, -2.500000000000000000 ) ) ;
#44467=DIRECTION ( 'NONE',  ( -0.000000000000000000, -0.000000000000000000, -1.000000000000000000 ) ) ;
#44487=VERTEX_POINT ( 'NONE', #35313 ) ;
#44512=ORIENTED_EDGE ( 'NONE', *, *, #16103, .T. ) ;
#44527=CARTESIAN_POINT ( 'NONE',  ( 18.80329974962065265, -105.8248132807389084, 5.500000000000000000 ) ) ;
#44529=DIRECTION ( 'NONE',  ( -0.8541291221503275466, 0.5200609990132993854, 0.000000000000000000 ) ) ;
#44537=CARTESIAN_POINT ( 'NONE',  ( -10.21100092698785033, -95.54625877152835756, -2.500000000000000000 ) ) ;
#44542=EDGE_CURVE ( 'NONE', #39825, #38904, #7143, .T. ) ;
#44547=VERTEX_POINT ( 'NONE', #22061 ) ;
#44548=EDGE_CURVE ( 'NONE', #25213, #45055, #40206, .T. ) ;
#44573=ORIENTED_EDGE ( 'NONE', *, *, #35671, .F. ) ;
#44597=EDGE_CURVE ( 'NONE', #47873, #14947, #29655, .T. ) ;
#44599=LINE ( 'NONE', #25990, #16913 ) ;
#44602=CARTESIAN_POINT ( 'NONE',  ( 0.000000000000000000, -89.50000000000000000, 2.500000000000000000 ) ) ;
#44610=CARTESIAN_POINT ( 'NONE',  ( 103.9230484541331947, -179.9999999999990337, 5.500000000000000000 ) ) ;
#44626=CARTESIAN_POINT ( 'NONE',  ( 12.13205353604972991, -140.1820037904669789, 5.500000000000000000 ) ) ;
#44636=CARTESIAN_POINT ( 'NONE',  ( -10.43921258969510824, -98.89258801967538659, 5.500000000000000000 ) ) ;
#44641=ORIENTED_EDGE ( 'NONE', *, *, #29733, .F. ) ;
#44642=EDGE_CURVE ( 'NONE', #21754, #35739, #27204, .T. ) ;
#44645=CARTESIAN_POINT ( 'NONE',  ( -17.26469406256017791, -140.1601175325492648, 5.500000000000000000 ) ) ;
#44651=DIRECTION ( 'NONE',  ( -0.8225049752423776450, -0.5687579148473765889, 0.000000000000000000 ) ) ;
#44653=DIRECTION ( 'NONE',  ( 0.6064928550163511956, 0.7950889364178798102, -0.000000000000000000 ) ) ;
#44657=EDGE_CURVE ( 'NONE', #3694, #21639, #8351, .T. ) ;
#44663=CARTESIAN_POINT ( 'NONE',  ( -18.24502636017238899, -100.7225776329765665, 5.500000000000000000 ) ) ;
#44677=PLANE ( 'NONE',  #1129 ) ;
#44681=LINE ( 'NONE', #25350, #36713 ) ;
#44682=ORIENTED_EDGE ( 'NONE', *, *, #48241, .T. ) ;
#44686=AXIS2_PLACEMENT_3D ( 'NONE', #6552, #4345, #37616 ) ;
#44688=FACE_BOUND ( 'NONE', #15705, .T. ) ;
#44700=FACE_OUTER_BOUND ( 'NONE', #17045, .T. ) ;
#44703=CARTESIAN_POINT ( 'NONE',  ( -22.67106064244953245, -113.6342314410295842, 5.500000000000000000 ) ) ;
#44705=LINE ( 'NONE', #47884, #7661 ) ;
#44716=DIRECTION ( 'NONE',  ( -0.000000000000000000, -0.000000000000000000, -1.000000000000000000 ) ) ;
#44718=DIRECTION ( 'NONE',  ( -0.2867529058022021404, 0.9580045777625456616, 0.000000000000000000 ) ) ;
#44724=FACE_OUTER_BOUND ( 'NONE', #33067, .T. ) ;
#44725=CARTESIAN_POINT ( 'NONE',  ( 1.355716935723751293, -120.6418968688129496, -2.500000000000000000 ) ) ;
#44726=ORIENTED_EDGE ( 'NONE', *, *, #38239, .T. ) ;
#44739=ADVANCED_FACE ( 'NONE', ( #23512 ), #30396, .F. ) ;
#44750=VECTOR ( 'NONE', #31935, 1000.000000000000227 ) ;
#44774=DIRECTION ( 'NONE',  ( -0.2867529058022035837, 0.9580045777625452175, 0.000000000000000000 ) ) ;
#44776=DIRECTION ( 'NONE',  ( -0.2306669878475648139, -0.9730327541852491491, 0.000000000000000000 ) ) ;
#44780=DIRECTION ( 'NONE',  ( 1.000000000000000000, 0.000000000000000000, 0.000000000000000000 ) ) ;
#44781=DIRECTION ( 'NONE',  ( -0.000000000000000000, -0.000000000000000000, -1.000000000000000000 ) ) ;
#44784=PRODUCT_DEFINITION_CONTEXT ( 'detailed design', #32577, 'design' ) ;
#44786=CARTESIAN_POINT ( 'NONE',  ( -22.53294031248082163, -134.0273518838794757, 5.500000000000000000 ) ) ;
#44802=AXIS2_PLACEMENT_3D ( 'NONE', #4571, #45936, #19714 ) ;
#44807=VERTEX_POINT ( 'NONE', #46777 ) ;
#44812=LINE ( 'NONE', #11297, #24390 ) ;
#44821=PLANE ( 'NONE',  #36794 ) ;
#44834=ADVANCED_FACE ( 'NONE', ( #1734 ), #27942, .F. ) ;
#44842=CARTESIAN_POINT ( 'NONE',  ( 24.95699195200416654, -110.9640411295978595, 5.500000000000000000 ) ) ;
#44852=ORIENTED_EDGE ( 'NONE', *, *, #36951, .F. ) ;
#44872=PLANE ( 'NONE',  #20706 ) ;
#44898=CARTESIAN_POINT ( 'NONE',  ( -4.653126046682595884, -146.1313684676804314, -5.500000000000000000 ) ) ;
#44905=LINE ( 'NONE', #598, #37206 ) ;
#44906=EDGE_CURVE ( 'NONE', #47208, #42659, #34772, .T. ) ;
#44915=DIRECTION ( 'NONE',  ( -0.000000000000000000, -0.000000000000000000, -1.000000000000000000 ) ) ;
#44927=ORIENTED_EDGE ( 'NONE', *, *, #23426, .F. ) ;
#44928=VECTOR ( 'NONE', #35858, 1000.000000000000000 ) ;
#44934=VERTEX_POINT ( 'NONE', #47949 ) ;
#44936=ORIENTED_EDGE ( 'NONE', *, *, #32986, .F. ) ;
#44939=CARTESIAN_POINT ( 'NONE',  ( -24.50849501662245800, -109.8101191361138831, -2.500000000000000444 ) ) ;
#44961=AXIS2_PLACEMENT_3D ( 'NONE', #25328, #31990, #46901 ) ;
#44971=LINE ( 'NONE', #45441, #9120 ) ;
#44973=EDGE_CURVE ( 'NONE', #21860, #30240, #14681, .T. ) ;
#44982=ADVANCED_FACE ( 'NONE', ( #33018 ), #29596, .F. ) ;
#44984=ORIENTED_EDGE ( 'NONE', *, *, #23829, .T. ) ;
#44985=DIRECTION ( 'NONE',  ( 0.8225049752423776450, 0.5687579148473765889, 0.000000000000000000 ) ) ;
#45004=CARTESIAN_POINT ( 'NONE',  ( -8.826826895187510402, -94.96827758698185562, -5.500000000000000000 ) ) ;
#45009=LINE ( 'NONE', #4385, #15074 ) ;
#45016=ORIENTED_EDGE ( 'NONE', *, *, #28562, .T. ) ;
#45021=CARTESIAN_POINT ( 'NONE',  ( -11.59517495878806947, -96.12423995607481686, -2.500000000000000000 ) ) ;
#45032=AXIS2_PLACEMENT_3D ( 'NONE', #39498, #6434, #21606 ) ;
#45041=VECTOR ( 'NONE', #17436, 1000.000000000000000 ) ;
#45055=VERTEX_POINT ( 'NONE', #36218 ) ;
#45061=DIRECTION ( 'NONE',  ( -0.3311129884571280546, -0.9435911131814402886, 0.000000000000000000 ) ) ;
#45089=CARTESIAN_POINT ( 'NONE',  ( -25.50183398199384754, -112.6408924756582053, 5.500000000000000000 ) ) ;
#45092=CARTESIAN_POINT ( 'NONE',  ( 0.000000000000000000, -89.50000000000000000, -2.500000000000000000 ) ) ;
#45094=DIRECTION ( 'NONE',  ( 0.000000000000000000, -0.000000000000000000, 1.000000000000000000 ) ) ;
#45105=VECTOR ( 'NONE', #7581, 1000.000000000000114 ) ;
#45107=VERTEX_POINT ( 'NONE', #45021 ) ;
#45110=VECTOR ( 'NONE', #40999, 1000.000000000000114 ) ;
#45118=CARTESIAN_POINT ( 'NONE',  ( -20.62008904684763166, -131.2721749321093512, 2.500000000000000000 ) ) ;
#45129=VERTEX_POINT ( 'NONE', #15635 ) ;
#45130=DIRECTION ( 'NONE',  ( -0.7585478161175706058, -0.6516173805718078471, 0.000000000000000000 ) ) ;
#45143=PLANE ( 'NONE',  #7474 ) ;
#45146=CARTESIAN_POINT ( 'NONE',  ( -19.90058851926621131, -132.5883508287165853, 5.500000000000000000 ) ) ;
#45159=EDGE_LOOP ( 'NONE', ( #8455, #20533, #38931, #48381 ) ) ;
#45165=VECTOR ( 'NONE', #29648, 1000.000000000000000 ) ;
#45166=EDGE_CURVE ( 'NONE', #31729, #21754, #34462, .T. ) ;
#45185=ORIENTED_EDGE ( 'NONE', *, *, #8302, .F. ) ;
#45192=DIRECTION ( 'NONE',  ( 0.000000000000000000, 0.000000000000000000, 1.000000000000000000 ) ) ;
#45206=ADVANCED_FACE ( 'NONE', ( #26659 ), #30824, .F. ) ;
#45212=ADVANCED_FACE ( 'NONE', ( #22735 ), #25918, .F. ) ;
#45213=PLANE ( 'NONE',  #6788 ) ;
#45226=ORIENTED_EDGE ( 'NONE', *, *, #8780, .F. ) ;
#45238=VERTEX_POINT ( 'NONE', #13176 ) ;
#45243=LINE ( 'NONE', #7562, #974 ) ;
#45256=CARTESIAN_POINT ( 'NONE',  ( -26.53422223201112828, -120.6595836127786043, 5.500000000000000000 ) ) ;
#45278=FACE_OUTER_BOUND ( 'NONE', #20719, .T. ) ;
#45302=EDGE_CURVE ( 'NONE', #29936, #5335, #23700, .T. ) ;
#45315=CARTESIAN_POINT ( 'NONE',  ( -23.97194136764370498, -131.3950000906648938, -5.500000000000000000 ) ) ;
#45326=ORIENTED_EDGE ( 'NONE', *, *, #29672, .F. ) ;
#45341=ORIENTED_EDGE ( 'NONE', *, *, #22409, .F. ) ;
#45346=CARTESIAN_POINT ( 'NONE',  ( -7.670864526094549163, -97.73662565058241114, 5.500000000000000000 ) ) ;
#45368=CARTESIAN_POINT ( 'NONE',  ( 19.29194287201271507, -133.5026271600380880, -2.500000000000000000 ) ) ;
#45393=ORIENTED_EDGE ( 'NONE', *, *, #22409, .T. ) ;
#45400=LINE ( 'NONE', #23610, #23075 ) ;
#45405=EDGE_LOOP ( 'NONE', ( #28189, #6168, #4596, #3205 ) ) ;
#45408=CARTESIAN_POINT ( 'NONE',  ( -0.8815729230226008184, -93.47222532549339746, 5.500000000000000000 ) ) ;
#45418=DIRECTION ( 'NONE',  ( -0.9781476007338069101, 0.2079116908177532363, 0.000000000000000000 ) ) ;
#45419=CARTESIAN_POINT ( 'NONE',  ( 6.377742925735834234, -145.7647898336708181, 5.500000000000000000 ) ) ;
#45420=CARTESIAN_POINT ( 'NONE',  ( -10.43921258969510824, -98.89258801967538659, -2.500000000000000000 ) ) ;
#45428=VECTOR ( 'NONE', #36041, 999.9999999999998863 ) ;
#45441=CARTESIAN_POINT ( 'NONE',  ( -14.87942725330654348, -141.9795960975983178, 5.500000000000000000 ) ) ;
#45449=ORIENTED_EDGE ( 'NONE', *, *, #8963, .F. ) ;
#45450=ORIENTED_EDGE ( 'NONE', *, *, #12109, .F. ) ;
#45481=DIRECTION ( 'NONE',  ( 0.1276937514489679404, 0.9918136447140103451, 0.000000000000000000 ) ) ;
#45493=EDGE_CURVE ( 'NONE', #7237, #41154, #41711, .T. ) ;
#45495=CARTESIAN_POINT ( 'NONE',  ( 11.41210121379328335, -99.40233154247455616, 2.500000000000000000 ) ) ;
#45500=AXIS2_PLACEMENT_3D ( 'NONE', #25079, #28050, #13846 ) ;
#45508=VERTEX_POINT ( 'NONE', #18930 ) ;
#45513=EDGE_CURVE ( 'NONE', #33738, #42694, #34844, .T. ) ;
#45518=VECTOR ( 'NONE', #30406, 1000.000000000000114 ) ;
#45537=VECTOR ( 'NONE', #16302, 1000.000000000000114 ) ;
#45543=DIRECTION ( 'NONE',  ( -0.1850432970638667129, 0.9827303690289281857, 0.000000000000000000 ) ) ;
#45547=CARTESIAN_POINT ( 'NONE',  ( 21.07894319797337701, -103.8699611390234878, 5.500000000000000000 ) ) ;
#45550=DIRECTION ( 'NONE',  ( -0.9435911131814398445, 0.3311129884571295534, 0.000000000000000000 ) ) ;
#45579=PLANE ( 'NONE',  #3440 ) ;
#45614=VECTOR ( 'NONE', #43290, 1000.000000000000000 ) ;
#45624=LINE ( 'NONE', #41719, #31760 ) ;
#45627=PLANE ( 'NONE',  #47215 ) ;
#45655=EDGE_CURVE ( 'NONE', #41264, #47615, #42924, .T. ) ;
#45664=ORIENTED_EDGE ( 'NONE', *, *, #44542, .T. ) ;
#45669=DIRECTION ( 'NONE',  ( -0.000000000000000000, -0.000000000000000000, -1.000000000000000000 ) ) ;
#45679=ORIENTED_EDGE ( 'NONE', *, *, #4651, .T. ) ;
#45683=PLANE ( 'NONE',  #16806 ) ;
#45688=CARTESIAN_POINT ( 'NONE',  ( -17.26469406256017791, -140.1601175325492648, -5.500000000000000000 ) ) ;
#45725=VECTOR ( 'NONE', #30427, 1000.000000000000114 ) ;
#45732=CARTESIAN_POINT ( 'NONE',  ( 14.59956846177685996, -138.4757300459248484, 2.500000000000000000 ) ) ;
#45754=DIRECTION ( 'NONE',  ( -0.000000000000000000, -0.000000000000000000, 1.000000000000000000 ) ) ;
#45756=EDGE_LOOP ( 'NONE', ( #9158, #20139, #32903, #14518 ) ) ;
#45763=ORIENTED_EDGE ( 'NONE', *, *, #11593, .T. ) ;
#45764=VECTOR ( 'NONE', #8146, 1000.000000000000227 ) ;
#45771=CARTESIAN_POINT ( 'NONE',  ( 8.700667342345820288, -98.11853780484867116, 5.500000000000000000 ) ) ;
#45781=ORIENTED_EDGE ( 'NONE', *, *, #46716, .F. ) ;
#45782=EDGE_LOOP ( 'NONE', ( #45798, #15847, #30269, #18620 ) ) ;
#45783=ORIENTED_EDGE ( 'NONE', *, *, #20504, .F. ) ;
#45788=CARTESIAN_POINT ( 'NONE',  ( -7.670864526094549163, -97.73662565058241114, 5.500000000000000000 ) ) ;
#45789=EDGE_LOOP ( 'NONE', ( #37811, #4497, #1654, #27636 ) ) ;
#45798=ORIENTED_EDGE ( 'NONE', *, *, #11147, .F. ) ;
#45809=CARTESIAN_POINT ( 'NONE',  ( 14.59956846177685996, -138.4757300459248484, 5.500000000000000000 ) ) ;
#45817=DIRECTION ( 'NONE',  ( -0.000000000000000000, -0.000000000000000000, -1.000000000000000000 ) ) ;
#45859=CARTESIAN_POINT ( 'NONE',  ( 26.28306158492127764, -123.3838844133976522, 2.500000000000000000 ) ) ;
#45860=CARTESIAN_POINT ( 'NONE',  ( 19.29194287201271862, -133.5026271600380880, 5.500000000000000000 ) ) ;
#45866=ORIENTED_EDGE ( 'NONE', *, *, #21379, .T. ) ;
#45868=DIRECTION ( 'NONE',  ( -0.000000000000000000, -0.000000000000000000, -1.000000000000000000 ) ) ;
#45869=FACE_OUTER_BOUND ( 'NONE', #39402, .T. ) ;
#45876=CARTESIAN_POINT ( 'NONE',  ( -21.67772167707813935, -110.8034581014852762, 5.500000000000000000 ) ) ;
#45880=LINE ( 'NONE', #31439, #3662 ) ;
#45898=ORIENTED_EDGE ( 'NONE', *, *, #38925, .T. ) ;
#45920=DIRECTION ( 'NONE',  ( 0.3853207896976533209, -0.9227826878668545785, 0.000000000000000000 ) ) ;
#45921=CARTESIAN_POINT ( 'NONE',  ( -22.53294031248082163, -134.0273518838794757, 5.500000000000000000 ) ) ;
#45929=CARTESIAN_POINT ( 'NONE',  ( 21.85433023846371370, -135.0628101570779620, -2.500000000000000444 ) ) ;
#45934=CARTESIAN_POINT ( 'NONE',  ( 22.08297821871651934, -111.8242998470044540, 5.500000000000000000 ) ) ;
#45936=DIRECTION ( 'NONE',  ( 0.2306669878475623159, 0.9730327541852497042, -0.000000000000000000 ) ) ;
#45944=CARTESIAN_POINT ( 'NONE',  ( 8.700667342345820288, -98.11853780484867116, 5.500000000000000000 ) ) ;
#45956=ORIENTED_EDGE ( 'NONE', *, *, #22803, .T. ) ;
#45959=CARTESIAN_POINT ( 'NONE',  ( 26.09152095774781799, -124.8716048804687375, -2.500000000000000444 ) ) ;
#45962=EDGE_CURVE ( 'NONE', #17038, #12299, #18874, .T. ) ;
#45971=VERTEX_POINT ( 'NONE', #23520 ) ;
#45974=DIRECTION ( 'NONE',  ( -0.7273375899149793211, 0.6862798483830554463, 0.000000000000000000 ) ) ;
#45976=EDGE_CURVE ( 'NONE', #30136, #1874, #19590, .T. ) ;
#45986=CARTESIAN_POINT ( 'NONE',  ( -23.97194136764370853, -131.3950000906648938, 2.500000000000000000 ) ) ;
#45988=DIRECTION ( 'NONE',  ( -0.000000000000000000, -0.000000000000000000, -1.000000000000000000 ) ) ;
#46006=VERTEX_POINT ( 'NONE', #45315 ) ;
#46007=EDGE_CURVE ( 'NONE', #12589, #37461, #26485, .T. ) ;
#46022=ADVANCED_FACE ( 'NONE', ( #12290 ), #42136, .F. ) ;
#46028=FACE_OUTER_BOUND ( 'NONE', #27846, .T. ) ;
#46033=ORIENTED_EDGE ( 'NONE', *, *, #44906, .T. ) ;
#46036=CARTESIAN_POINT ( 'NONE',  ( 14.59956846177685996, -138.4757300459248484, 5.500000000000000000 ) ) ;
#46037=LINE ( 'NONE', #6125, #18799 ) ;
#46044=ORIENTED_EDGE ( 'NONE', *, *, #39969, .T. ) ;
#46052=EDGE_CURVE ( 'NONE', #24556, #35257, #8112, .T. ) ;
#46058=CARTESIAN_POINT ( 'NONE',  ( 23.11608002360578240, -124.4885236261218182, 5.500000000000000000 ) ) ;
#46063=LINE ( 'NONE', #769, #21756 ) ;
#46080=ORIENTED_EDGE ( 'NONE', *, *, #6587, .T. ) ;
#46086=FACE_OUTER_BOUND ( 'NONE', #40667, .T. ) ;
#46087=EDGE_CURVE ( 'NONE', #45129, #37535, #32090, .T. ) ;
#46090=DIRECTION ( 'NONE',  ( 0.000000000000000000, 0.000000000000000000, 1.000000000000000000 ) ) ;
#46117=CARTESIAN_POINT ( 'NONE',  ( -3.961125083139900749, -143.2122702051246677, -2.500000000000000000 ) ) ;
#46132=VECTOR ( 'NONE', #42953, 1000.000000000000000 ) ;
#46135=EDGE_CURVE ( 'NONE', #11806, #14848, #43347, .T. ) ;
#46143=ORIENTED_EDGE ( 'NONE', *, *, #2298, .F. ) ;
#46155=ADVANCED_FACE ( 'NONE', ( #2218 ), #46539, .F. ) ;
#46166=CARTESIAN_POINT ( 'NONE',  ( -19.90058851926621131, -132.5883508287165853, 5.500000000000000000 ) ) ;
#46167=ORIENTED_EDGE ( 'NONE', *, *, #43863, .F. ) ;
#46184=AXIS2_PLACEMENT_3D ( 'NONE', #11317, #30159, #37245 ) ;
#46189=EDGE_CURVE ( 'NONE', #25478, #5822, #47010, .T. ) ;
#46193=EDGE_LOOP ( 'NONE', ( #3911, #27114, #43299, #3644 ) ) ;
#46222=ORIENTED_EDGE ( 'NONE', *, *, #33705, .F. ) ;
#46233=CARTESIAN_POINT ( 'NONE',  ( 25.81725066941077529, -113.8380548628854854, 5.500000000000000000 ) ) ;
#46237=ORIENTED_EDGE ( 'NONE', *, *, #33819, .T. ) ;
#46242=ORIENTED_EDGE ( 'NONE', *, *, #20173, .F. ) ;
#46251=DIRECTION ( 'NONE',  ( 0.5687579148473744795, -0.8225049752423790883, 0.000000000000000000 ) ) ;
#46252=VECTOR ( 'NONE', #11037, 1000.000000000000000 ) ;
#46256=ORIENTED_EDGE ( 'NONE', *, *, #1620, .T. ) ;
#46285=CYLINDRICAL_SURFACE ( 'NONE', #31266, 32.50000000000000000 ) ;
#46292=VECTOR ( 'NONE', #30322, 1000.000000000000114 ) ;
#46303=PRODUCT_CONTEXT ( 'NONE', #10722, 'mechanical' ) ;
#46314=VECTOR ( 'NONE', #8415, 1000.000000000000000 ) ;
#46322=ORIENTED_EDGE ( 'NONE', *, *, #17606, .F. ) ;
#46334=CARTESIAN_POINT ( 'NONE',  ( -30.50000000000000000, -120.0000000000000000, -2.500000000000000000 ) ) ;
#46361=EDGE_CURVE ( 'NONE', #5936, #18083, #25506, .T. ) ;
#46368=CARTESIAN_POINT ( 'NONE',  ( 0.6180191030787338669, -93.50720753887522108, 2.500000000000000000 ) ) ;
#46389=ORIENTED_EDGE ( 'NONE', *, *, #35139, .F. ) ;
#46390=DIRECTION ( 'NONE',  ( -1.000000000000000000, 0.000000000000000000, -0.000000000000000000 ) ) ;
#46394=AXIS2_PLACEMENT_3D ( 'NONE', #1755, #20585, #20843 ) ;
#46395=CARTESIAN_POINT ( 'NONE',  ( -1.355716935723729089, -119.3581031311870362, -2.500000000000000000 ) ) ;
#46397=DIRECTION ( 'NONE',  ( -0.1276937514489679404, -0.9918136447140103451, 0.000000000000000000 ) ) ;
#46407=CARTESIAN_POINT ( 'NONE',  ( 70.53423027509757048, -217.0820393249931044, -5.500000000000000000 ) ) ;
#46417=EDGE_LOOP ( 'NONE', ( #46857, #36943 ) ) ;
#46420=DIRECTION ( 'NONE',  ( -0.7273375899149802093, 0.6862798483830544471, 0.000000000000000000 ) ) ;
#46442=ORIENTED_EDGE ( 'NONE', *, *, #28247, .T. ) ;
#46447=EDGE_CURVE ( 'NONE', #2793, #28062, #15644, .T. ) ;
#46461=VECTOR ( 'NONE', #18447, 1000.000000000000114 ) ;
#46463=ADVANCED_FACE ( 'NONE', ( #19069 ), #480, .F. ) ;
#46464=ORIENTED_EDGE ( 'NONE', *, *, #14026, .F. ) ;
#46468=LINE ( 'NONE', #31065, #36040 ) ;
#46470=VECTOR ( 'NONE', #47962, 1000.000000000000114 ) ;
#46490=( LENGTH_UNIT ( ) NAMED_UNIT ( * ) SI_UNIT ( .MILLI., .METRE. ) );
#46494=AXIS2_PLACEMENT_3D ( 'NONE', #41742, #23608, #38550 ) ;
#46499=ORIENTED_EDGE ( 'NONE', *, *, #27644, .F. ) ;
#46518=ORIENTED_EDGE ( 'NONE', *, *, #44657, .T. ) ;
#46536=CARTESIAN_POINT ( 'NONE',  ( 5.822613034544236399, -142.8165987265839760, 5.500000000000000000 ) ) ;
#46539=PLANE ( 'NONE',  #35688 ) ;
#46552=ORIENTED_EDGE ( 'NONE', *, *, #15266, .F. ) ;
#46570=LINE ( 'NONE', #38252, #6310 ) ;
#46576=CARTESIAN_POINT ( 'NONE',  ( 2.047646702416564768, -96.54137380445985173, 5.500000000000000000 ) ) ;
#46581=CARTESIAN_POINT ( 'NONE',  ( 0.000000000000000000, -120.0000000000000000, 2.500000000000000000 ) ) ;
#46595=PLANE ( 'NONE',  #31621 ) ;
#46613=ORIENTED_EDGE ( 'NONE', *, *, #10394, .F. ) ;
#46614=CARTESIAN_POINT ( 'NONE',  ( 6.377742925735834234, -145.7647898336708181, -5.500000000000000000 ) ) ;
#46627=CARTESIAN_POINT ( 'NONE',  ( 21.07894319797337701, -103.8699611390234878, 5.500000000000000000 ) ) ;
#46631=VERTEX_POINT ( 'NONE', #35452 ) ;
#46647=LINE ( 'NONE', #31237, #40968 ) ;
#46650=ADVANCED_FACE ( 'NONE', ( #6806 ), #13905, .F. ) ;
#46662=CARTESIAN_POINT ( 'NONE',  ( 20.07203437053270179, -132.2214334768125354, -2.500000000000000000 ) ) ;
#46671=ADVANCED_FACE ( 'NONE', ( #18039 ), #25870, .T. ) ;
#46691=VERTEX_POINT ( 'NONE', #25390 ) ;
#46706=CARTESIAN_POINT ( 'NONE',  ( 2.117611129180199558, -93.54218975225703048, -2.500000000000000444 ) ) ;
#46711=ORIENTED_EDGE ( 'NONE', *, *, #2641, .F. ) ;
#46716=EDGE_CURVE ( 'NONE', #15261, #5216, #21233, .T. ) ;
#46719=VERTEX_POINT ( 'NONE', #47193 ) ;
#46722=DIRECTION ( 'NONE',  ( -0.000000000000000000, -0.000000000000000000, -1.000000000000000000 ) ) ;
#46736=VERTEX_POINT ( 'NONE', #24916 ) ;
#46741=CARTESIAN_POINT ( 'NONE',  ( -22.67106064244953245, -113.6342314410295842, 5.500000000000000000 ) ) ;
#46775=CARTESIAN_POINT ( 'NONE',  ( 23.41451323550360186, -132.5004227906269989, 2.500000000000000000 ) ) ;
#46777=CARTESIAN_POINT ( 'NONE',  ( 3.429551818649054340, -146.3199197248623875, 5.500000000000000000 ) ) ;
#46778=DIRECTION ( 'NONE',  ( -0.8225049752423791993, -0.5687579148473745905, 0.000000000000000000 ) ) ;
#46792=ORIENTED_EDGE ( 'NONE', *, *, #38670, .F. ) ;
#46806=ADVANCED_FACE ( 'NONE', ( #8250 ), #18761, .F. ) ;
#46833=CARTESIAN_POINT ( 'NONE',  ( -15.44521549751111422, -137.7748507232956001, 5.500000000000000000 ) ) ;
#46836=DIRECTION ( 'NONE',  ( 0.6516173805718078471, -0.7585478161175706058, 0.000000000000000000 ) ) ;
#46843=LINE ( 'NONE', #8907, #7387 ) ;
#46854=CARTESIAN_POINT ( 'NONE',  ( 23.11608002360578240, -124.4885236261218182, -5.500000000000000000 ) ) ;
#46856=ORIENTED_EDGE ( 'NONE', *, *, #14821, .T. ) ;
#46857=ORIENTED_EDGE ( 'NONE', *, *, #28735, .T. ) ;
#46859=PLANE ( 'NONE',  #31566 ) ;
#46867=ORIENTED_EDGE ( 'NONE', *, *, #23829, .F. ) ;
#46897=DIRECTION ( 'NONE',  ( -0.000000000000000000, -0.000000000000000000, -1.000000000000000000 ) ) ;
#46901=DIRECTION ( 'NONE',  ( -0.8090169943749426773, -0.5877852522924797984, 0.000000000000000000 ) ) ;
#46903=DIRECTION ( 'NONE',  ( 0.1850432970638656582, -0.9827303690289285187, 0.000000000000000000 ) ) ;
#46913=EDGE_CURVE ( 'NONE', #42101, #21999, #27572, .T. ) ;
#46914=VECTOR ( 'NONE', #22035, 1000.000000000000114 ) ;
#46921=VERTEX_POINT ( 'NONE', #1626 ) ;
#46922=ORIENTED_EDGE ( 'NONE', *, *, #12757, .T. ) ;
#46964=ORIENTED_EDGE ( 'NONE', *, *, #3767, .T. ) ;
#46965=ORIENTED_EDGE ( 'NONE', *, *, #18827, .T. ) ;
#46989=CARTESIAN_POINT ( 'NONE',  ( 1.474095553543393056, -119.7224350544041869, -2.500000000000000000 ) ) ;
#46991=ORIENTED_EDGE ( 'NONE', *, *, #10947, .T. ) ;
#46996=CARTESIAN_POINT ( 'NONE',  ( 22.63442173698368620, -133.7816164738524378, -2.500000000000000000 ) ) ;
#47001=EDGE_LOOP ( 'NONE', ( #5218, #36565, #25268, #2358 ) ) ;
#47006=DIRECTION ( 'NONE',  ( 0.000000000000000000, 0.000000000000000000, 1.000000000000000000 ) ) ;
#47010=LINE ( 'NONE', #5183, #41143 ) ;
#47011=LINE ( 'NONE', #35753, #27793 ) ;
#47015=LINE ( 'NONE', #35987, #32681 ) ;
#47016=DIRECTION ( 'NONE',  ( -0.9827303690289285187, -0.1850432970638656860, 0.000000000000000000 ) ) ;
#47042=DIRECTION ( 'NONE',  ( -0.000000000000000000, -0.000000000000000000, -1.000000000000000000 ) ) ;
#47044=ORIENTED_EDGE ( 'NONE', *, *, #15862, .F. ) ;
#47058=VECTOR ( 'NONE', #28630, 1000.000000000000114 ) ;
#47072=DIRECTION ( 'NONE',  ( -0.1045284632676570929, 0.9945218953682730678, 0.000000000000000000 ) ) ;
#47098=LINE ( 'NONE', #28026, #46132 ) ;
#47101=CARTESIAN_POINT ( 'NONE',  ( 0.000000000000000000, -120.0000000000000000, -2.500000000000000000 ) ) ;
#47102=CARTESIAN_POINT ( 'NONE',  ( 23.49916127795269460, -121.5130826919798039, -5.500000000000000000 ) ) ;
#47106=CARTESIAN_POINT ( 'NONE',  ( 16.84844760790522855, -103.5491698323862124, -5.500000000000000000 ) ) ;
#47110=CARTESIAN_POINT ( 'NONE',  ( -0.8815729230226008184, -93.47222532549339746, -5.500000000000000000 ) ) ;
#47124=EDGE_CURVE ( 'NONE', #33083, #9793, #6979, .T. ) ;
#47157=EDGE_LOOP ( 'NONE', ( #20234, #6595, #35585, #12304 ) ) ;
#47166=FACE_OUTER_BOUND ( 'NONE', #39561, .T. ) ;
#47170=FACE_BOUND ( 'NONE', #13484, .T. ) ;
#47188=EDGE_CURVE ( 'NONE', #2793, #13936, #17752, .T. ) ;
#47193=CARTESIAN_POINT ( 'NONE',  ( -13.05994868825747446, -139.5943292883446532, 2.500000000000000000 ) ) ;
#47198=VECTOR ( 'NONE', #24208, 1000.000000000000114 ) ;
#47208=VERTEX_POINT ( 'NONE', #30230 ) ;
#47213=VECTOR ( 'NONE', #35569, 1000.000000000000114 ) ;
#47215=AXIS2_PLACEMENT_3D ( 'NONE', #601, #355, #16022 ) ;
#47237=VERTEX_POINT ( 'NONE', #15053 ) ;
#47250=DIRECTION ( 'NONE',  ( 0.000000000000000000, 0.000000000000000000, 1.000000000000000000 ) ) ;
#47264=ADVANCED_FACE ( 'NONE', ( #3785 ), #48331, .F. ) ;
#47274=VECTOR ( 'NONE', #10701, 1000.000000000000114 ) ;
#47284=DIRECTION ( 'NONE',  ( 0.9435911131814395114, -0.3311129884571304971, 0.000000000000000000 ) ) ;
#47316=CARTESIAN_POINT ( 'NONE',  ( 2.117611129180199558, -93.54218975225703048, 2.500000000000000000 ) ) ;
#47320=EDGE_CURVE ( 'NONE', #4369, #20259, #29730, .T. ) ;
#47323=AXIS2_PLACEMENT_3D ( 'NONE', #11010, #7815, #22742 ) ;
#47339=ADVANCED_BREP_SHAPE_REPRESENTATION ( '', ( #19421, #11636 ), #10062 ) ;
#47353=ORIENTED_EDGE ( 'NONE', *, *, #27356, .T. ) ;
#47361=VERTEX_POINT ( 'NONE', #5664 ) ;
#47362=FACE_OUTER_BOUND ( 'NONE', #17496, .T. ) ;
#47381=AXIS2_PLACEMENT_3D ( 'NONE', #42185, #23836, #4743 ) ;
#47384=DIRECTION ( 'NONE',  ( -0.000000000000000000, -0.000000000000000000, -1.000000000000000000 ) ) ;
#47410=VERTEX_POINT ( 'NONE', #21060 ) ;
#47412=ORIENTED_EDGE ( 'NONE', *, *, #39640, .T. ) ;
#47414=FACE_BOUND ( 'NONE', #24792, .T. ) ;
#47419=SURFACE_STYLE_FILL_AREA ( #32496 ) ;
#47423=ORIENTED_EDGE ( 'NONE', *, *, #25793, .T. ) ;
#47442=ORIENTED_EDGE ( 'NONE', *, *, #30848, .F. ) ;
#47476=ORIENTED_EDGE ( 'NONE', *, *, #1090, .F. ) ;
#47493=ORIENTED_EDGE ( 'NONE', *, *, #17073, .T. ) ;
#47500=ORIENTED_EDGE ( 'NONE', *, *, #45493, .F. ) ;
#47501=EDGE_CURVE ( 'NONE', #22663, #24556, #21295, .T. ) ;
#47504=EDGE_CURVE ( 'NONE', #28861, #36901, #44304, .T. ) ;
#47528=DIRECTION ( 'NONE',  ( -0.4796670183876294291, 0.8774505977381983346, 0.000000000000000000 ) ) ;
#47533=CARTESIAN_POINT ( 'NONE',  ( 0.1915406271734537980, -118.5122795329289858, 2.500000000000000000 ) ) ;
#47539=CARTESIAN_POINT ( 'NONE',  ( 0.000000000000000000, -120.0000000000000000, 5.500000000000000000 ) ) ;
#47548=VECTOR ( 'NONE', #29671, 1000.000000000000000 ) ;
#47564=EDGE_CURVE ( 'NONE', #5271, #47208, #3413, .T. ) ;
#47571=CARTESIAN_POINT ( 'NONE',  ( 0.5480546763151027401, -96.50639159107802811, -2.500000000000000000 ) ) ;
#47575=ORIENTED_EDGE ( 'NONE', *, *, #24155, .T. ) ;
#47578=ORIENTED_EDGE ( 'NONE', *, *, #11621, .F. ) ;
#47597=FACE_OUTER_BOUND ( 'NONE', #15190, .T. ) ;
#47602=DIRECTION ( 'NONE',  ( 0.6862798483830533369, 0.7273375899149812085, -0.000000000000000000 ) ) ;
#47615=VERTEX_POINT ( 'NONE', #37681 ) ;
#47626=LINE ( 'NONE', #14108, #14892 ) ;
#47630=LINE ( 'NONE', #14112, #44393 ) ;
#47652=CARTESIAN_POINT ( 'NONE',  ( 0.1915406271734537980, -118.5122795329289858, -2.500000000000000000 ) ) ;
#47658=LINE ( 'NONE', #2884, #26252 ) ;
#47665=EDGE_CURVE ( 'NONE', #22663, #2423, #22517, .T. ) ;
#47668=EDGE_CURVE ( 'NONE', #34199, #14963, #38170, .T. ) ;
#47671=EDGE_CURVE ( 'NONE', #20465, #43248, #4412, .T. ) ;
#47691=LINE ( 'NONE', #3645, #12542 ) ;
#47703=CARTESIAN_POINT ( 'NONE',  ( 20.85212586905262100, -130.9402397935870965, 5.500000000000000000 ) ) ;
#47727=ADVANCED_FACE ( 'NONE', ( #18821 ), #15180, .F. ) ;
#47736=ORIENTED_EDGE ( 'NONE', *, *, #17472, .F. ) ;
#47743=LINE ( 'NONE', #9840, #1920 ) ;
#47752=ORIENTED_EDGE ( 'NONE', *, *, #39973, .T. ) ;
#47754=DIRECTION ( 'NONE',  ( -0.8774505977381983346, -0.4796670183876294291, 0.000000000000000000 ) ) ;
#47761=VERTEX_POINT ( 'NONE', #22746 ) ;
#47764=LINE ( 'NONE', #41184, #21201 ) ;
#47767=LINE ( 'NONE', #18144, #26272 ) ;
#47768=ADVANCED_FACE ( 'NONE', ( #34240 ), #30577, .F. ) ;
#47785=EDGE_LOOP ( 'NONE', ( #35738, #30964, #16179, #19154 ) ) ;
#47788=CARTESIAN_POINT ( 'NONE',  ( 11.41210121379327980, -99.40233154247455616, -2.500000000000000000 ) ) ;
#47789=EDGE_LOOP ( 'NONE', ( #35045, #14242, #14713, #36801 ) ) ;
#47798=VECTOR ( 'NONE', #32026, 1000.000000000000114 ) ;
#47822=DIRECTION ( 'NONE',  ( -0.000000000000000000, -0.000000000000000000, -1.000000000000000000 ) ) ;
#47827=ORIENTED_EDGE ( 'NONE', *, *, #13792, .T. ) ;
#47858=VECTOR ( 'NONE', #20019, 1000.000000000000000 ) ;
#47860=ORIENTED_EDGE ( 'NONE', *, *, #8776, .F. ) ;
#47871=ORIENTED_EDGE ( 'NONE', *, *, #47564, .T. ) ;
#47873=VERTEX_POINT ( 'NONE', #40790 ) ;
#47884=CARTESIAN_POINT ( 'NONE',  ( -6.880223345695647197, -142.5202692415819854, -5.500000000000000000 ) ) ;
#47898=AXIS2_PLACEMENT_3D ( 'NONE', #2223, #10282, #32786 ) ;
#47916=EDGE_CURVE ( 'NONE', #43886, #36733, #15565, .T. ) ;
#47917=PLANE ( 'NONE',  #1489 ) ;
#47941=ORIENTED_EDGE ( 'NONE', *, *, #24413, .T. ) ;
#47949=CARTESIAN_POINT ( 'NONE',  ( -14.87942725330654348, -141.9795960975983178, -5.500000000000000000 ) ) ;
#47956=CARTESIAN_POINT ( 'NONE',  ( 22.94323693612312809, -114.6983135802921083, -5.500000000000000000 ) ) ;
#47961=CARTESIAN_POINT ( 'NONE',  ( 9.984461079971730157, -95.40710393340120277, 5.500000000000000000 ) ) ;
#47962=DIRECTION ( 'NONE',  ( -0.3311129884571281101, -0.9435911131814402886, 0.000000000000000000 ) ) ;
#47965=EDGE_LOOP ( 'NONE', ( #3578, #33185 ) ) ;
#47973=LINE ( 'NONE', #44068, #27667 ) ;
#47974=ORIENTED_EDGE ( 'NONE', *, *, #29855, .F. ) ;
#47978=VECTOR ( 'NONE', #1444, 1000.000000000000114 ) ;
#47982=ORIENTED_EDGE ( 'NONE', *, *, #35139, .T. ) ;
#47991=ADVANCED_FACE ( 'NONE', ( #11657 ), #42480, .F. ) ;
#48017=ADVANCED_FACE ( 'NONE', ( #397 ), #4072, .F. ) ;
#48025=CARTESIAN_POINT ( 'NONE',  ( 30.50000000000000000, -120.0000000000000000, 5.500000000000000888 ) ) ;
#48037=FACE_OUTER_BOUND ( 'NONE', #6416, .T. ) ;
#48039=DIRECTION ( 'NONE',  ( -0.9038112904824853189, 0.4279312458752977943, 0.000000000000000000 ) ) ;
#48065=AXIS2_PLACEMENT_3D ( 'NONE', #9, #44087, #40654 ) ;
#48087=ORIENTED_EDGE ( 'NONE', *, *, #35646, .T. ) ;
#48100=DIRECTION ( 'NONE',  ( -0.000000000000000000, -0.000000000000000000, -1.000000000000000000 ) ) ;
#48116=EDGE_CURVE ( 'NONE', #17971, #37535, #36767, .T. ) ;
#48123=DIRECTION ( 'NONE',  ( -0.9918136447140101231, 0.1276937514489694114, 0.000000000000000000 ) ) ;
#48130=ORIENTED_EDGE ( 'NONE', *, *, #39640, .F. ) ;
#48157=DIRECTION ( 'NONE',  ( -0.9435911131814402886, 0.3311129884571281101, 0.000000000000000000 ) ) ;
#48162=EDGE_LOOP ( 'NONE', ( #33787, #20079, #18966, #8104 ) ) ;
#48175=AXIS2_PLACEMENT_3D ( 'NONE', #16201, #38724, #24743 ) ;
#48201=DIRECTION ( 'NONE',  ( 0.7585478161175716050, 0.6516173805718067369, 0.000000000000000000 ) ) ;
#48220=CARTESIAN_POINT ( 'NONE',  ( 0.000000000000000000, -120.0000000000000000, 2.500000000000000000 ) ) ;
#48225=ORIENTED_EDGE ( 'NONE', *, *, #45976, .T. ) ;
#48241=EDGE_CURVE ( 'NONE', #44547, #34735, #46063, .T. ) ;
#48246=PLANE ( 'NONE',  #19668 ) ;
#48257=EDGE_LOOP ( 'NONE', ( #19647, #2436, #724, #42600 ) ) ;
#48259=FACE_OUTER_BOUND ( 'NONE', #43368, .T. ) ;
#48266=FACE_OUTER_BOUND ( 'NONE', #29373, .T. ) ;
#48281=ORIENTED_EDGE ( 'NONE', *, *, #21305, .F. ) ;
#48294=CARTESIAN_POINT ( 'NONE',  ( -21.33958957442910886, -129.9559990355020034, 5.500000000000000000 ) ) ;
#48295=LINE ( 'NONE', #40969, #41815 ) ;
#48310=ORIENTED_EDGE ( 'NONE', *, *, #36423, .F. ) ;
#48322=FACE_OUTER_BOUND ( 'NONE', #12255, .T. ) ;
#48329=CARTESIAN_POINT ( 'NONE',  ( 19.12409105625795291, -101.5943176906707919, -5.500000000000000000 ) ) ;
#48331=PLANE ( 'NONE',  #44337 ) ;
#48344=ADVANCED_FACE ( 'NONE', ( #13022 ), #5422, .T. ) ;
#48352=CARTESIAN_POINT ( 'NONE',  ( 16.84844760790522855, -103.5491698323862124, 5.500000000000000000 ) ) ;
#48353=ORIENTED_EDGE ( 'NONE', *, *, #38140, .T. ) ;
#48364=ORIENTED_EDGE ( 'NONE', *, *, #34252, .T. ) ;
#48366=EDGE_LOOP ( 'NONE', ( #34803, #15837, #41454, #27133 ) ) ;
#48368=VECTOR ( 'NONE', #42823, 1000.000000000000000 ) ;
#48381=ORIENTED_EDGE ( 'NONE', *, *, #29672, .T. ) ;
#48391=DIRECTION ( 'NONE',  ( 0.8774505977381983346, 0.4796670183876293736, 0.000000000000000000 ) ) ;
#48404=EDGE_LOOP ( 'NONE', ( #13044, #46222, #29408, #21785 ) ) ;
#48405=ADVANCED_FACE ( 'NONE', ( #32330 ), #16919, .F. ) ;
#48408=ORIENTED_EDGE ( 'NONE', *, *, #19482, .T. ) ;
#48413=EDGE_LOOP ( 'NONE', ( #12352, #39873, #43032, #2048 ) ) ;
#48432=DIRECTION ( 'NONE',  ( -0.5687579148473743684, 0.8225049752423791993, 0.000000000000000000 ) ) ;
#48437=LINE ( 'NONE', #7580, #21869 ) ;
ENDSEC;
END-ISO-10303-21;
